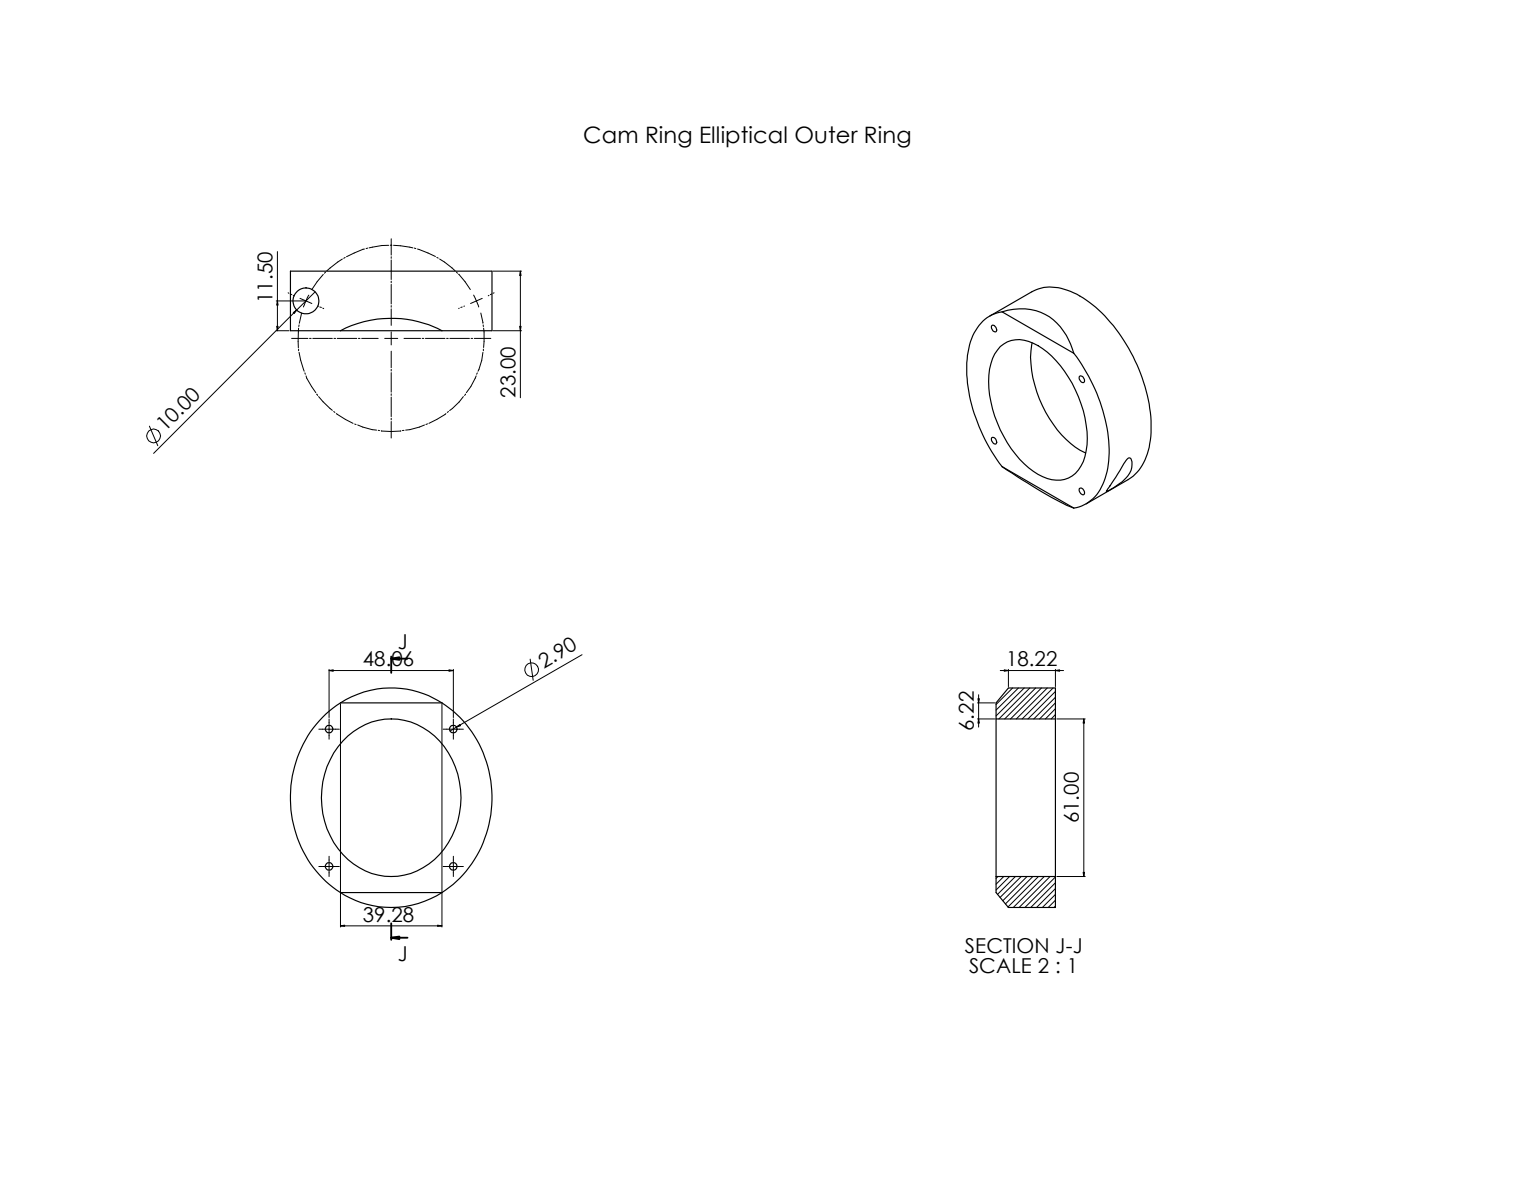
ISO-10303-21;
HEADER;
FILE_DESCRIPTION (('STEP AP214'),
    '1' );
FILE_NAME ('Cam Ring Elliptical Outer Ring.step',
    '2026-10-18T20:16:25',
    ( '' ),
    ( '' ),
    'SwSTEP 2.0',
    'SolidWorks 2025',
    '' );
FILE_SCHEMA (( 'AUTOMOTIVE_DESIGN' ));
ENDSEC;

DATA;
#6=ADVANCED_FACE ( 'NONE', ( #26858 ), #19364, .F. ) ;
#7=CARTESIAN_POINT ( 'NONE',  ( -10.18506332983503881, -29.04537757311073065, 24.50000000000000000 ) ) ;
#35=EDGE_CURVE ( 'NONE', #21045, #27073, #21273, .T. ) ;
#67=ORIENTED_EDGE ( 'NONE', *, *, #8805, .T. ) ;
#72=LINE ( 'NONE', #9585, #22578 ) ;
#83=EDGE_LOOP ( 'NONE', ( #20575, #9372 ) ) ;
#262=CARTESIAN_POINT ( 'NONE',  ( 37.01111991330344608, -13.41299137855487977, 15.98316150592440543 ) ) ;
#276=FACE_BOUND ( 'NONE', #21490, .T. ) ;
#306=CARTESIAN_POINT ( 'NONE',  ( -19.18576292979354392, -22.55620591602727742, 1.500000000000001332 ) ) ;
#358=ORIENTED_EDGE ( 'NONE', *, *, #1752, .T. ) ;
#391=DIRECTION ( 'NONE',  ( 0.000000000000000000, 0.000000000000000000, 1.000000000000000000 ) ) ;
#417=DIRECTION ( 'NONE',  ( 0.000000000000000000, -0.6368814469962913449, -0.7709617516270896864 ) ) ;
#463=CARTESIAN_POINT ( 'NONE',  ( -28.06941827521502475, 29.50589912660750969, 12.07342606168410093 ) ) ;
#502=AXIS2_PLACEMENT_3D ( 'NONE', #13971, #30353, #16313 ) ;
#521=ORIENTED_EDGE ( 'NONE', *, *, #17753, .F. ) ;
#566=AXIS2_PLACEMENT_3D ( 'NONE', #22892, #22733, #8869 ) ;
#617=EDGE_CURVE ( 'NONE', #17587, #16446, #72, .T. ) ;
#647=CARTESIAN_POINT ( 'NONE',  ( 30.67761959283033235, -26.24282937179839337, 17.43639551542309718 ) ) ;
#664=ORIENTED_EDGE ( 'NONE', *, *, #18976, .F. ) ;
#674=CARTESIAN_POINT ( 'NONE',  ( -35.78636641679163688, 16.94032250535760653, 17.18098098232441018 ) ) ;
#680=DIRECTION ( 'NONE',  ( 1.000000000000000000, 0.000000000000000000, -0.000000000000000000 ) ) ;
#716=CARTESIAN_POINT ( 'NONE',  ( 32.98805937973595093, -22.67054169308931222, 8.000000000000003553 ) ) ;
#724=DIRECTION ( 'NONE',  ( -1.000000000000000000, 0.000000000000000000, 0.000000000000000000 ) ) ;
#774=PRODUCT_DEFINITION_CONTEXT ( 'detailed design', #23710, 'design' ) ;
#782=CARTESIAN_POINT ( 'NONE',  ( -24.03057240117690441, -26.57182937991348481, 1.500000000000001332 ) ) ;
#787=ADVANCED_FACE ( 'NONE', ( #2872, #12396, #22043, #15022, #21896, #10048 ), #19557, .T. ) ;
#799=EDGE_CURVE ( 'NONE', #24988, #12790, #28615, .T. ) ;
#813=CARTESIAN_POINT ( 'NONE',  ( 32.98805937973593672, 0.000000000000000000, 18.00000000000000000 ) ) ;
#820=EDGE_LOOP ( 'NONE', ( #21441, #11766, #4890, #26992 ) ) ;
#826=CARTESIAN_POINT ( 'NONE',  ( -37.62287076735433544, 11.19774653192125591, 14.88367311033162821 ) ) ;
#857=VECTOR ( 'NONE', #15365, 1000.000000000000000 ) ;
#888=CARTESIAN_POINT ( 'NONE',  ( -12.17697269691152329, 40.41958668078866879, 21.44088211123782983 ) ) ;
#909=CARTESIAN_POINT ( 'NONE',  ( 22.58267429318971864, 26.57182937991349903, 26.54355021145562787 ) ) ;
#923=CARTESIAN_POINT ( 'NONE',  ( -29.80493885133978083, 27.41358096823880786, 9.131458560479140729 ) ) ;
#947=CARTESIAN_POINT ( 'NONE',  ( 10.18506332983505303, 29.04537757311072710, 24.50000000000000000 ) ) ;
#969=CARTESIAN_POINT ( 'NONE',  ( 30.16810946264573445, -26.93506237724814412, 17.13185035612489315 ) ) ;
#992=CARTESIAN_POINT ( 'NONE',  ( -33.31304828179383293, 22.10896115714093924, 8.000000000000005329 ) ) ;
#1038=B_SPLINE_CURVE_WITH_KNOTS ( 'NONE', 3,
 ( #18272, #27795, #6420, #16082, #4219, #6712, #9365, #28701, #30717, #14183 ),
 .UNSPECIFIED., .F., .F.,
 ( 4, 2, 2, 2, 4 ),
 ( 0.000000000000000000, 0.005347349928980100683, 0.01069469985796020657, 0.01604204978694031072, 0.02138939971592041661 ),
 .UNSPECIFIED. ) ;
#1042=DIRECTION ( 'NONE',  ( -0.000000000000000000, -1.000000000000000000, -0.000000000000000000 ) ) ;
#1119=CARTESIAN_POINT ( 'NONE',  ( 29.78864511397301484, -27.43196031439082461, 9.154089586762928832 ) ) ;
#1134=DIRECTION ( 'NONE',  ( 1.000000000000000000, 0.000000000000000000, 0.000000000000000000 ) ) ;
#1140=CARTESIAN_POINT ( 'NONE',  ( 10.18506332983505303, 29.04537757311072710, 1.500000000000000000 ) ) ;
#1141=CARTESIAN_POINT ( 'NONE',  ( -34.21431199717225979, 20.40874709909905604, 8.143388502677929353 ) ) ;
#1200=ADVANCED_FACE ( 'NONE', ( #23844 ), #2488, .F. ) ;
#1234=CARTESIAN_POINT ( 'NONE',  ( -19.64177907938615064, -36.71644397333972876, 24.50000000000000000 ) ) ;
#1267=AXIS2_PLACEMENT_3D ( 'NONE', #10644, #30128, #8758 ) ;
#1278=CARTESIAN_POINT ( 'NONE',  ( 31.30424506559346298, -25.35202612174932568, 8.284888684157436956 ) ) ;
#1298=CARTESIAN_POINT ( 'NONE',  ( -6.192647045995789412, -41.97176936070047049, 20.15864424522374065 ) ) ;
#1299=CARTESIAN_POINT ( 'NONE',  ( -37.98074266006555888, 9.653107878580014400, 13.30882976141995222 ) ) ;
#1359=AXIS2_PLACEMENT_3D ( 'NONE', #12045, #21538, #28424 ) ;
#1413=CARTESIAN_POINT ( 'NONE',  ( -10.18506332983504237, -29.04537757311072710, 1.500000000000000000 ) ) ;
#1419=( GEOMETRIC_REPRESENTATION_CONTEXT ( 3 ) GLOBAL_UNCERTAINTY_ASSIGNED_CONTEXT ( ( #17991 ) ) GLOBAL_UNIT_ASSIGNED_CONTEXT ( ( #21477, #23197, #28368 ) ) REPRESENTATION_CONTEXT ( 'NONE', 'WORKASPACE' ) );
#1422=AXIS2_PLACEMENT_3D ( 'NONE', #15991, #2089, #3991 ) ;
#1507=DIRECTION ( 'NONE',  ( 0.000000000000000000, 0.000000000000000000, -1.000000000000000000 ) ) ;
#1534=CARTESIAN_POINT ( 'NONE',  ( -25.47847050916410439, -26.57182937991348481, 24.50000000000000000 ) ) ;
#1568=CARTESIAN_POINT ( 'NONE',  ( -25.47847050916410439, -26.57182937991348481, 26.54355021145562787 ) ) ;
#1615=CARTESIAN_POINT ( 'NONE',  ( -18.94750032487069902, -37.15750911010949409, 24.13564184353800712 ) ) ;
#1683=CYLINDRICAL_SURFACE ( 'NONE', #566, 4.999999999999997335 ) ;
#1690=CARTESIAN_POINT ( 'NONE',  ( -28.54661976619838981, 28.95749706969278847, 15.30506458469658071 ) ) ;
#1697=DIRECTION ( 'NONE',  ( -0.000000000000000000, -0.000000000000000000, -1.000000000000000000 ) ) ;
#1752=EDGE_CURVE ( 'NONE', #8742, #20574, #14920, .T. ) ;
#1753=DIRECTION ( 'NONE',  ( 1.000000000000000000, 0.000000000000000000, 0.000000000000000000 ) ) ;
#1759=CARTESIAN_POINT ( 'NONE',  ( -27.75715622479468081, 2.303929616531696922E-16, 24.50000000000000000 ) ) ;
#1865=AXIS2_PLACEMENT_3D ( 'NONE', #30712, #18883, #7020 ) ;
#1895=CARTESIAN_POINT ( 'NONE',  ( 19.64177907938615064, 36.71644397333972876, 24.50000000000000000 ) ) ;
#1911=CARTESIAN_POINT ( 'NONE',  ( -25.48568755041063838, 12.36160011285429583, 24.50000000000000000 ) ) ;
#1956=CARTESIAN_POINT ( 'NONE',  ( 3.395021109945021376, 30.50000000000000000, 24.50000000000000000 ) ) ;
#1962=ORIENTED_EDGE ( 'NONE', *, *, #2846, .F. ) ;
#2032=FACE_OUTER_BOUND ( 'NONE', #19721, .T. ) ;
#2089=DIRECTION ( 'NONE',  ( 0.000000000000000000, -1.000000000000000000, 0.000000000000000000 ) ) ;
#2101=CARTESIAN_POINT ( 'NONE',  ( 14.50629223094009035, 39.46103756294984777, 22.23272703466988887 ) ) ;
#2123=ORIENTED_EDGE ( 'NONE', *, *, #24038, .F. ) ;
#2132=EDGE_CURVE ( 'NONE', #24759, #6184, #9736, .T. ) ;
#2139=CARTESIAN_POINT ( 'NONE',  ( 32.98805937973593672, 0.000000000000000000, 13.00000000000000178 ) ) ;
#2156=FACE_BOUND ( 'NONE', #12173, .T. ) ;
#2217=CARTESIAN_POINT ( 'NONE',  ( 24.03057240117691862, 26.57182937991349903, 26.54355021145562787 ) ) ;
#2302=FACE_OUTER_BOUND ( 'NONE', #17026, .T. ) ;
#2381=EDGE_CURVE ( 'NONE', #17270, #19224, #29354, .T. ) ;
#2415=CARTESIAN_POINT ( 'NONE',  ( 32.98805937973593672, 0.000000000000000000, 13.00000000000000178 ) ) ;
#2420=CARTESIAN_POINT ( 'NONE',  ( 0.000000000000000000, 36.71644397333972165, 24.50000000000000000 ) ) ;
#2488=CYLINDRICAL_SURFACE ( 'NONE', #20811, 1.447898107987198646 ) ;
#2505=CARTESIAN_POINT ( 'NONE',  ( -25.48568755041063838, 12.36160011285429583, 24.50000000000000000 ) ) ;
#2608=CARTESIAN_POINT ( 'NONE',  ( 36.63885979765411349, -14.57625097221031751, 16.42869143197607684 ) ) ;
#2614=ORIENTED_EDGE ( 'NONE', *, *, #22128, .T. ) ;
#2732=DIRECTION ( 'NONE',  ( 1.000000000000000000, 0.000000000000000000, 0.000000000000000000 ) ) ;
#2765=CARTESIAN_POINT ( 'NONE',  ( 37.87340355726868779, -10.14209321046124934, 14.07067178332522239 ) ) ;
#2798=CARTESIAN_POINT ( 'NONE',  ( -30.18521284010790851, 26.91230962269908034, 8.856508891382476989 ) ) ;
#2846=EDGE_CURVE ( 'NONE', #25535, #4436, #15712, .T. ) ;
#2854=DIRECTION ( 'NONE',  ( -0.000000000000000000, -0.000000000000000000, -1.000000000000000000 ) ) ;
#2872=FACE_BOUND ( 'NONE', #7887, .T. ) ;
#2919=CARTESIAN_POINT ( 'NONE',  ( -22.58267429318971864, 26.57182937991348481, 26.54355021145562787 ) ) ;
#2939=ORIENTED_EDGE ( 'NONE', *, *, #28576, .F. ) ;
#2966=CARTESIAN_POINT ( 'NONE',  ( -28.10697575488836364, 29.46351030971690932, 14.10614635148330898 ) ) ;
#3002=CARTESIAN_POINT ( 'NONE',  ( 29.54181686732680845, -27.74713163033052865, 9.373611838719332567 ) ) ;
#3016=EDGE_LOOP ( 'NONE', ( #29920, #15554 ) ) ;
#3031=DIRECTION ( 'NONE',  ( 0.000000000000000000, 0.000000000000000000, 1.000000000000000000 ) ) ;
#3068=PLANE ( 'NONE',  #24267 ) ;
#3069=CARTESIAN_POINT ( 'NONE',  ( 37.79362409831109915, -10.49224821554092735, 11.60540311995022833 ) ) ;
#3151=CARTESIAN_POINT ( 'NONE',  ( 30.28907500942318620, -26.77591773196712310, 8.779599968084907502 ) ) ;
#3173=DIRECTION ( 'NONE',  ( 1.000000000000000000, 0.000000000000000000, 0.000000000000000000 ) ) ;
#3177=CARTESIAN_POINT ( 'NONE',  ( -37.98866957712698422, 9.615774924837397819, 13.14437204739174447 ) ) ;
#3216=CARTESIAN_POINT ( 'NONE',  ( -3.469446951953614189E-15, -30.50000000000000711, 1.500000000000000000 ) ) ;
#3220=CARTESIAN_POINT ( 'NONE',  ( 37.66982319287888004, -11.00826088415979775, 11.23380626198473387 ) ) ;
#3225=ORIENTED_EDGE ( 'NONE', *, *, #3454, .F. ) ;
#3227=CARTESIAN_POINT ( 'NONE',  ( -7.114862909856333850, 41.83185039483213075, 20.27422947789757046 ) ) ;
#3228=CARTESIAN_POINT ( 'NONE',  ( -48.64405085385531180, 18.29172496293576344, 24.50000000000000355 ) ) ;
#3252=CARTESIAN_POINT ( 'NONE',  ( -32.98805937973593672, 22.67054169308932288, 8.000000000000003553 ) ) ;
#3277=CARTESIAN_POINT ( 'NONE',  ( 25.48568755041062417, 12.36160011285428872, 1.500000000000001332 ) ) ;
#3324=CARTESIAN_POINT ( 'NONE',  ( 10.18506332983503349, -29.04537757311073420, 1.500000000000000000 ) ) ;
#3325=CARTESIAN_POINT ( 'NONE',  ( -37.98737094879278686, 9.621865500938454829, 12.81607210702588340 ) ) ;
#3358=ORIENTED_EDGE ( 'NONE', *, *, #26402, .F. ) ;
#3438=DIRECTION ( 'NONE',  ( 0.000000000000000000, 0.000000000000000000, 1.000000000000000000 ) ) ;
#3440=CARTESIAN_POINT ( 'NONE',  ( 3.469446951953614189E-15, 30.50000000000000000, 24.50000000000000000 ) ) ;
#3454=EDGE_CURVE ( 'NONE', #16680, #16446, #9263, .T. ) ;
#3482=CARTESIAN_POINT ( 'NONE',  ( 24.03057240117690441, -26.57182937991349903, 1.500000000000001332 ) ) ;
#3489=CARTESIAN_POINT ( 'NONE',  ( 25.48568755041062417, 12.36160011285428872, 1.500000000000000000 ) ) ;
#3543=VERTEX_POINT ( 'NONE', #10112 ) ;
#3597=VERTEX_POINT ( 'NONE', #22890 ) ;
#3640=CARTESIAN_POINT ( 'NONE',  ( -37.48217255283579874, 11.74471995787475187, 15.19832840420940734 ) ) ;
#3646=CARTESIAN_POINT ( 'NONE',  ( 2.168404344971008868E-16, 30.50000000000000000, 24.50000000000000000 ) ) ;
#3698=CARTESIAN_POINT ( 'NONE',  ( 22.58267429318970443, -26.57182937991349903, 26.54355021145562787 ) ) ;
#3701=ADVANCED_FACE ( 'NONE', ( #18676 ), #20697, .F. ) ;
#3759=( BOUNDED_SURFACE ( )  B_SPLINE_SURFACE ( 3, 1, ( 
 ( #4545, #13914 ),
 ( #6734, #16245 ),
 ( #25916, #11431 ),
 ( #4855, #16401 ) ),
 .UNSPECIFIED., .F., .F., .T. ) 
 B_SPLINE_SURFACE_WITH_KNOTS ( ( 4, 4 ),
 ( 2, 2 ),
 ( 0.000000000000000000, 1.000000000000000000 ),
 ( 0.000000000000000000, 1.000000000000000000 ),
 .UNSPECIFIED. ) 
 GEOMETRIC_REPRESENTATION_ITEM ( )  RATIONAL_B_SPLINE_SURFACE ( (
 ( 1.000000000000000000, 1.000000000000000000),
 ( 0.3333333333333333703, 0.3333333333333333703),
 ( 0.3333333333333333703, 0.3333333333333333703),
 ( 1.000000000000000000, 1.000000000000000000) ) ) 
 REPRESENTATION_ITEM ( '' )  SURFACE ( )  );
#3881=EDGE_CURVE ( 'NONE', #8417, #14704, #23959, .T. ) ;
#3883=CARTESIAN_POINT ( 'NONE',  ( -22.58267429318970443, -26.57182937991348481, 26.54355021145562787 ) ) ;
#3889=CARTESIAN_POINT ( 'NONE',  ( -29.41946345040754096, 27.90099610680150377, 16.50653305109835500 ) ) ;
#3912=FACE_OUTER_BOUND ( 'NONE', #27376, .T. ) ;
#3970=B_SPLINE_CURVE_WITH_KNOTS ( 'NONE', 3,
 ( #19233, #18949, #16589, #19088, #4896, #19696, #674, #10502, #8494, #25001, #13156, #22037, #3640, #826, #10350, #29221, #29532, #20328, #7860, #1299, #3177, #3325, #12856, #17369, #29853, #22648, #24683, #22495, #24531, #27043, #15483, #19862, #10814, #20163, #29380, #8020, #8169, #17522, #1141, #5824, #992, #26729 ),
 .UNSPECIFIED., .F., .F.,
 ( 4, 2, 2, 2, 2, 2, 2, 2, 2, 2, 2, 2, 2, 2, 2, 2, 2, 2, 2, 2, 4 ),
 ( 0.02151600789256482779, 0.02343308447725669583, 0.02535016106194856386, 0.02918431423133229299, 0.03110139081602415062, 0.03301846740071601172, 0.03397700569306194573, 0.03493554398540787975, 0.03589408227775381377, 0.03637335142392678078, 0.03685262057009974779, 0.03733188971627271480, 0.03781115886244568874, 0.03876969715479162970, 0.03972823544713757066, 0.04068677373948351161, 0.04260385032417539353, 0.04452092690886727544, 0.04835508007825103927, 0.05027215666294292118, 0.05218923324763480309 ),
 .UNSPECIFIED. ) ;
#3991=DIRECTION ( 'NONE',  ( 0.000000000000000000, 0.000000000000000000, 1.000000000000000000 ) ) ;
#4029=FACE_OUTER_BOUND ( 'NONE', #6532, .T. ) ;
#4056=ORIENTED_EDGE ( 'NONE', *, *, #35, .F. ) ;
#4135=PLANE ( 'NONE',  #1422 ) ;
#4150=CARTESIAN_POINT ( 'NONE',  ( -19.64177907938615064, -36.71644397333972876, 24.50000000000000000 ) ) ;
#4207=EDGE_CURVE ( 'NONE', #12790, #24988, #12731, .T. ) ;
#4219=CARTESIAN_POINT ( 'NONE',  ( 12.13957942244085331, -40.43335259791965086, 21.42951026665136993 ) ) ;
#4238=CIRCLE ( 'NONE', #1267, 1.447898107987198646 ) ;
#4346=EDGE_LOOP ( 'NONE', ( #5689, #11400, #10833, #14682 ) ) ;
#4354=CARTESIAN_POINT ( 'NONE',  ( 22.58267429318970443, -26.57182937991349903, 24.50000000000000000 ) ) ;
#4429=ADVANCED_FACE ( 'NONE', ( #18306 ), #16112, .F. ) ;
#4436=VERTEX_POINT ( 'NONE', #11440 ) ;
#4502=VERTEX_POINT ( 'NONE', #27662 ) ;
#4520=CARTESIAN_POINT ( 'NONE',  ( 32.98805937973592961, -22.67054169308934064, 18.00000000000000000 ) ) ;
#4545=CARTESIAN_POINT ( 'NONE',  ( -4.776122516674677878E-15, -42.50000000000000000, 24.50000000000000000 ) ) ;
#4781=CARTESIAN_POINT ( 'NONE',  ( 34.23529990058388250, -20.39752770391714876, 17.87601422035457333 ) ) ;
#4789=ORIENTED_EDGE ( 'NONE', *, *, #24819, .F. ) ;
#4848=UNCERTAINTY_MEASURE_WITH_UNIT (LENGTH_MEASURE( 1.000000000000000082E-05 ), #21403, 'distance_accuracy_value', 'NONE');
#4854=AXIS2_PLACEMENT_3D ( 'NONE', #29179, #19979, #7517 ) ;
#4855=CARTESIAN_POINT ( 'NONE',  ( 0.000000000000000000, 42.50000000000000000, 24.50000000000000000 ) ) ;
#4871=CARTESIAN_POINT ( 'NONE',  ( -22.58267429318970443, -26.57182937991348481, 24.50000000000000000 ) ) ;
#4890=ORIENTED_EDGE ( 'NONE', *, *, #3454, .T. ) ;
#4896=CARTESIAN_POINT ( 'NONE',  ( -34.50378612593421224, 19.82132163181573148, 17.77334831411353733 ) ) ;
#4913=ORIENTED_EDGE ( 'NONE', *, *, #16059, .F. ) ;
#4915=CARTESIAN_POINT ( 'NONE',  ( -3.469446951953614189E-15, -30.50000000000000711, 24.50000000000000000 ) ) ;
#4947=CARTESIAN_POINT ( 'NONE',  ( 37.94146307560947662, -9.835134691610786462, 13.69354701980937961 ) ) ;
#4961=FACE_BOUND ( 'NONE', #30357, .T. ) ;
#5020=CYLINDRICAL_SURFACE ( 'NONE', #1359, 1.447898107987198646 ) ;
#5032=ADVANCED_FACE ( 'NONE', ( #8064 ), #3068, .F. ) ;
#5038=CIRCLE ( 'NONE', #21514, 1.447898107987198646 ) ;
#5040=AXIS2_PLACEMENT_3D ( 'NONE', #16169, #25068, #25684 ) ;
#5077=CYLINDRICAL_SURFACE ( 'NONE', #10597, 1.447898107987198646 ) ;
#5133=ORIENTED_EDGE ( 'NONE', *, *, #13621, .T. ) ;
#5150=CARTESIAN_POINT ( 'NONE',  ( 24.03057240117690441, -26.57182937991349903, 24.50000000000000000 ) ) ;
#5199=PRODUCT ( 'Cam Ring Elliptical Outer Ring', 'Cam Ring Elliptical Outer Ring', '', ( #24403 ) ) ;
#5204=ADVANCED_FACE ( 'NONE', ( #5871 ), #23001, .F. ) ;
#5207=CARTESIAN_POINT ( 'NONE',  ( -3.469446951953614189E-15, -30.50000000000000711, 1.500000000000000000 ) ) ;
#5235=CARTESIAN_POINT ( 'NONE',  ( -22.58267429318970443, -26.57182937991348481, 1.500000000000001332 ) ) ;
#5256=CARTESIAN_POINT ( 'NONE',  ( 37.70070167288648122, -10.88189949536004342, 14.68280373647734116 ) ) ;
#5278=ORIENTED_EDGE ( 'NONE', *, *, #25507, .F. ) ;
#5290=CARTESIAN_POINT ( 'NONE',  ( -28.00213357088913924, 29.58171923439856243, 13.43815007647722659 ) ) ;
#5316=CARTESIAN_POINT ( 'NONE',  ( 77.99999999999998579, 42.50000000000000000, 1.500000000000000222 ) ) ;
#5332=CARTESIAN_POINT ( 'NONE',  ( 28.30074574513791674, -29.24255319736864323, 14.75302129891823988 ) ) ;
#5363=ORIENTED_EDGE ( 'NONE', *, *, #24082, .F. ) ;
#5455=CARTESIAN_POINT ( 'NONE',  ( -28.29454325412426030, 29.24967321222531780, 14.73627230915420583 ) ) ;
#5493=CARTESIAN_POINT ( 'NONE',  ( 32.52407683584942788, -23.45431533902839405, 17.97980913012589710 ) ) ;
#5574=CARTESIAN_POINT ( 'NONE',  ( -8.074094344234884818E-15, 42.50000000000000000, 19.72227980406325543 ) ) ;
#5600=B_SPLINE_CURVE_WITH_KNOTS ( 'NONE', 3,
 ( #16648, #26154, #4781, #23805, #24576, #8065, #12126, #17570, #2608, #262, #19745, #14756, #15062, #22082, #5256, #7448, #21781, #2765, #7597, #4947, #19446, #26943, #24428, #12592, #21627, #28962, #26789, #19918, #24276, #12278, #3069, #3220, #24116, #19292, #29432, #9775, #14459, #28811, #23961, #21934, #22242, #7916, #16951, #716 ),
 .UNSPECIFIED., .F., .F.,
 ( 4, 2, 2, 2, 2, 2, 2, 2, 2, 2, 2, 2, 2, 2, 2, 2, 2, 2, 2, 2, 2, 4 ),
 ( 6.938893903907228378E-18, 0.003866689226559128639, 0.005800033839838692959, 0.007733378453118257279, 0.009666723066397821598, 0.01160006767967738592, 0.01256673998631717241, 0.01353341229295695718, 0.01401674844627684956, 0.01450008459959674367, 0.01498342075291663779, 0.01522508882957658398, 0.01546675690623653190, 0.01595009305955642429, 0.01643342921287630973, 0.01740010151951609102, 0.01836677382615587231, 0.01933344613279565360, 0.02126679074607521619, 0.02320013535935478224, 0.02706682458591391088, 0.03093351381247303605 ),
 .UNSPECIFIED. ) ;
#5632=CARTESIAN_POINT ( 'NONE',  ( 19.18576292979354392, -22.55620591602728453, 1.500000000000001332 ) ) ;
#5689=ORIENTED_EDGE ( 'NONE', *, *, #25026, .F. ) ;
#5720=CARTESIAN_POINT ( 'NONE',  ( 24.03057240117690441, -26.57182937991349903, 26.54355021145562787 ) ) ;
#5730=ADVANCED_FACE ( 'NONE', ( #30600 ), #27828, .F. ) ;
#5762=ORIENTED_EDGE ( 'NONE', *, *, #20655, .F. ) ;
#5824=CARTESIAN_POINT ( 'NONE',  ( -33.62358953728911359, 21.54311338121501507, 8.031451707336353607 ) ) ;
#5853=CARTESIAN_POINT ( 'NONE',  ( -32.98805937973593672, 0.000000000000000000, 18.00000000000000000 ) ) ;
#5865=CARTESIAN_POINT ( 'NONE',  ( -32.98805937973593672, 80.00000000000000000, 8.000000000000003553 ) ) ;
#5871=FACE_OUTER_BOUND ( 'NONE', #7763, .T. ) ;
#5933=ORIENTED_EDGE ( 'NONE', *, *, #18705, .F. ) ;
#5983=DIRECTION ( 'NONE',  ( 0.000000000000000000, 0.000000000000000000, 1.000000000000000000 ) ) ;
#6062=CARTESIAN_POINT ( 'NONE',  ( -32.05743189141918492, 24.22168755390175576, 17.93996624350626590 ) ) ;
#6126=CARTESIAN_POINT ( 'NONE',  ( -12.13118772005164026, -40.43574026512624897, 21.42753784591547017 ) ) ;
#6184=VERTEX_POINT ( 'NONE', #27241 ) ;
#6236=CARTESIAN_POINT ( 'NONE',  ( 24.03057240117690441, -26.57182937991349903, 1.500000000000001332 ) ) ;
#6346=DIRECTION ( 'NONE',  ( 0.000000000000000000, -1.000000000000000000, 0.000000000000000000 ) ) ;
#6364=CIRCLE ( 'NONE', #26278, 1.447898107987198646 ) ;
#6380=CARTESIAN_POINT ( 'NONE',  ( -29.78995557804746497, 27.43027642362437390, 16.84702627303446221 ) ) ;
#6420=CARTESIAN_POINT ( 'NONE',  ( 16.79415820840736728, -38.40031270401642871, 23.10897800509315658 ) ) ;
#6426=CIRCLE ( 'NONE', #8442, 4.999999999999997335 ) ;
#6439=MECHANICAL_DESIGN_GEOMETRIC_PRESENTATION_REPRESENTATION('',(#19881),#14397);
#6444=CARTESIAN_POINT ( 'NONE',  ( -4.776122516674677878E-15, -42.50000000000000000, 19.72227980406325543 ) ) ;
#6498=ORIENTED_EDGE ( 'NONE', *, *, #26501, .T. ) ;
#6532=EDGE_LOOP ( 'NONE', ( #22804, #521, #30469, #26719 ) ) ;
#6555=ORIENTED_EDGE ( 'NONE', *, *, #2132, .T. ) ;
#6633=CARTESIAN_POINT ( 'NONE',  ( 10.18506332983503349, -29.04537757311073420, 24.50000000000000000 ) ) ;
#6712=CARTESIAN_POINT ( 'NONE',  ( 8.778767752581492445, -41.45290410434266448, 20.58727206569324153 ) ) ;
#6723=CARTESIAN_POINT ( 'NONE',  ( 19.64177907938615064, -36.71644397333972876, 24.50000000000000000 ) ) ;
#6734=CARTESIAN_POINT ( 'NONE',  ( 77.99999999999998579, -42.50000000000002132, 24.50000000000000000 ) ) ;
#6782=CARTESIAN_POINT ( 'NONE',  ( 1.794035659141604899, 42.46622758119957552, 19.75017875872448059 ) ) ;
#6789=FACE_OUTER_BOUND ( 'NONE', #820, .T. ) ;
#6801=VECTOR ( 'NONE', #27037, 1000.000000000000000 ) ;
#6845=PRODUCT_DEFINITION ( 'UNKNOWN', '', #8918, #774 ) ;
#6900=VECTOR ( 'NONE', #17424, 1000.000000000000000 ) ;
#7020=DIRECTION ( 'NONE',  ( -1.000000000000000000, 0.000000000000000000, 0.000000000000000000 ) ) ;
#7031=ORIENTED_EDGE ( 'NONE', *, *, #21011, .F. ) ;
#7175=CARTESIAN_POINT ( 'NONE',  ( 0.000000000000000000, 42.50000000000000000, 24.50000000000000000 ) ) ;
#7212=( NAMED_UNIT ( * ) PLANE_ANGLE_UNIT ( ) SI_UNIT ( $, .RADIAN. ) );
#7245=EDGE_CURVE ( 'NONE', #3543, #29877, #21049, .T. ) ;
#7344=CARTESIAN_POINT ( 'NONE',  ( -19.18576292979354392, -22.55620591602727742, 24.50000000000000000 ) ) ;
#7349=DIRECTION ( 'NONE',  ( 0.000000000000000000, 0.000000000000000000, 1.000000000000000000 ) ) ;
#7368=ORIENTED_EDGE ( 'NONE', *, *, #29806, .F. ) ;
#7396=AXIS2_PLACEMENT_3D ( 'NONE', #9486, #28514, #21014 ) ;
#7448=CARTESIAN_POINT ( 'NONE',  ( 37.79101548699587454, -10.50083399009356988, 14.39349168688145575 ) ) ;
#7498=CARTESIAN_POINT ( 'NONE',  ( -3.395021109945006721, -30.50000000000000711, 1.500000000000001332 ) ) ;
#7517=DIRECTION ( 'NONE',  ( 0.000000000000000000, 0.7709617516270895754, 0.6368814469962912339 ) ) ;
#7597=CARTESIAN_POINT ( 'NONE',  ( 37.89827105978137922, -10.03094553435206926, 13.95238484874844787 ) ) ;
#7634=CARTESIAN_POINT ( 'NONE',  ( -27.98709118423092690, 29.59858197539721658, 13.20579471836786745 ) ) ;
#7641=ADVANCED_FACE ( 'NONE', ( #26447 ), #5077, .F. ) ;
#7660=VECTOR ( 'NONE', #18726, 1000.000000000000000 ) ;
#7682=CARTESIAN_POINT ( 'NONE',  ( 27.98837345756654926, -29.59714202224856194, 13.23495098233264500 ) ) ;
#7688=EDGE_CURVE ( 'NONE', #26441, #20574, #18128, .T. ) ;
#7763=EDGE_LOOP ( 'NONE', ( #29336, #358, #5133, #5933 ) ) ;
#7782=CARTESIAN_POINT ( 'NONE',  ( -24.03057240117691862, 26.57182937991348481, 24.50000000000000000 ) ) ;
#7831=CARTESIAN_POINT ( 'NONE',  ( 32.40545545705547426, -23.64849546015198811, 17.96741959276885581 ) ) ;
#7837=AXIS2_PLACEMENT_3D ( 'NONE', #11186, #22716, #27884 ) ;
#7860=CARTESIAN_POINT ( 'NONE',  ( -37.95344354766306338, 9.779784673403119299, 13.60598863365600053 ) ) ;
#7864=DIRECTION ( 'NONE',  ( -0.000000000000000000, 1.000000000000000000, -0.000000000000000000 ) ) ;
#7887=EDGE_LOOP ( 'NONE', ( #5363, #4056 ) ) ;
#7916=CARTESIAN_POINT ( 'NONE',  ( 34.22030469044062073, -20.42639397296790804, 8.120957071897569435 ) ) ;
#7926=FACE_OUTER_BOUND ( 'NONE', #16867, .T. ) ;
#7952=DIRECTION ( 'NONE',  ( 1.000000000000000000, 0.000000000000000000, 0.000000000000000000 ) ) ;
#7998=CARTESIAN_POINT ( 'NONE',  ( 28.11261193835277084, -29.45712586627402985, 14.13030833143228371 ) ) ;
#8019=CARTESIAN_POINT ( 'NONE',  ( 27.75715622479469147, -6.315477654728063328E-15, 1.500000000000000000 ) ) ;
#8020=CARTESIAN_POINT ( 'NONE',  ( -35.77650053662277685, 16.96546617299160076, 8.812125201147090081 ) ) ;
#8059=LINE ( 'NONE', #5865, #857 ) ;
#8064=FACE_OUTER_BOUND ( 'NONE', #12470, .T. ) ;
#8065=CARTESIAN_POINT ( 'NONE',  ( 35.77999848792182291, -16.92214645512589755, 17.15740857515053364 ) ) ;
#8076=CYLINDRICAL_SURFACE ( 'NONE', #14140, 1.447898107987198646 ) ;
#8105=CARTESIAN_POINT ( 'NONE',  ( -30.31362811597099238, 26.74039424657907205, 8.772790042427574875 ) ) ;
#8119=B_SPLINE_CURVE_WITH_KNOTS ( 'NONE', 3,
 ( #15570, #28153, #6782, #10741, #13964, #20823, #23460, #17761, #8986, #23318, #2101, #18502, #11623, #18802 ),
 .UNSPECIFIED., .F., .F.,
 ( 4, 2, 2, 2, 2, 2, 4 ),
 ( 0.02129242833620984335, 0.02395618414067833199, 0.02661993994514682063, 0.03194745155408380138, 0.03461120735855229003, 0.03727496316302077867, 0.04260247477195776289 ),
 .UNSPECIFIED. ) ;
#8127=DIRECTION ( 'NONE',  ( -0.000000000000000000, -0.000000000000000000, -1.000000000000000000 ) ) ;
#8147=CARTESIAN_POINT ( 'NONE',  ( 31.04966398092921409, -25.72093259340003968, 8.382396669768365172 ) ) ;
#8169=CARTESIAN_POINT ( 'NONE',  ( -35.29666319828150023, 18.12171425783904866, 8.528199801003413683 ) ) ;
#8330=CARTESIAN_POINT ( 'NONE',  ( 32.98805937973593672, -80.00000000000000000, 13.00000000000000178 ) ) ;
#8344=ORIENTED_EDGE ( 'NONE', *, *, #15087, .T. ) ;
#8389=DIRECTION ( 'NONE',  ( 0.000000000000000000, 0.000000000000000000, 1.000000000000000000 ) ) ;
#8407=B_SPLINE_SURFACE_WITH_KNOTS ( 'NONE', 3, 1, ( 
 ( #20125, #29956 ),
 ( #29805, #17482 ),
 ( #13271, #27004 ),
 ( #15272, #5632 ),
 ( #24803, #29643 ),
 ( #15127, #8448 ),
 ( #24643, #3277 ),
 ( #17791, #12806 ),
 ( #947, #10459 ),
 ( #19973, #29492 ),
 ( #3440, #12961 ) ),
 .UNSPECIFIED., .F., .F., .F.,
 ( 4, 1, 1, 1, 1, 1, 1, 1, 4 ),
 ( 2, 2 ),
 ( 3.141592653589793116, 3.534291735288517255, 3.926990816987241395, 4.319689898685965090, 4.712388980384689674, 5.105088062083414258, 5.497787143782137953, 5.890486225480861648, 6.283185307179586232 ),
 ( 0.000000000000000000, 1.000000000000000000 ),
 .UNSPECIFIED. ) ;
#8417=VERTEX_POINT ( 'NONE', #9350 ) ;
#8442=AXIS2_PLACEMENT_3D ( 'NONE', #20677, #6346, #8389 ) ;
#8448=CARTESIAN_POINT ( 'NONE',  ( 27.75715622479469147, -6.315477654728063328E-15, 1.500000000000001332 ) ) ;
#8452=EDGE_CURVE ( 'NONE', #17270, #16132, #18072, .T. ) ;
#8458=CIRCLE ( 'NONE', #11942, 1.447898107987198646 ) ;
#8471=ADVANCED_FACE ( 'NONE', ( #4029 ), #1683, .F. ) ;
#8479=ORIENTED_EDGE ( 'NONE', *, *, #22585, .T. ) ;
#8494=CARTESIAN_POINT ( 'NONE',  ( -36.62615482024158098, 14.61410224498927946, 16.44210843200423255 ) ) ;
#8522=VERTEX_POINT ( 'NONE', #1234 ) ;
#8550=VERTEX_POINT ( 'NONE', #17925 ) ;
#8555=CARTESIAN_POINT ( 'NONE',  ( -19.64177907938615064, 36.71644397333972876, 24.50000000000000000 ) ) ;
#8568=DIRECTION ( 'NONE',  ( -0.000000000000000000, -0.000000000000000000, -1.000000000000000000 ) ) ;
#8583=CARTESIAN_POINT ( 'NONE',  ( 2.168404344971008868E-16, 30.50000000000000000, 1.500000000000000000 ) ) ;
#8639=CARTESIAN_POINT ( 'NONE',  ( -3.395021109945014270, 30.50000000000000355, 24.50000000000000000 ) ) ;
#8678=CARTESIAN_POINT ( 'NONE',  ( -3.469446951953614189E-15, -30.50000000000000711, 24.50000000000000000 ) ) ;
#8742=VERTEX_POINT ( 'NONE', #23960 ) ;
#8758=DIRECTION ( 'NONE',  ( 1.000000000000000000, 0.000000000000000000, 0.000000000000000000 ) ) ;
#8771=CARTESIAN_POINT ( 'NONE',  ( -13.72594918703051725, -39.82203247533167456, 21.93451384618056110 ) ) ;
#8791=B_SPLINE_CURVE_WITH_KNOTS ( 'NONE', 3,
 ( #6444, #20620, #11432, #1298, #22960, #20476, #27964, #6126, #8771, #8942, #27654, #17997, #1615, #25475 ),
 .UNSPECIFIED., .F., .F.,
 ( 4, 2, 2, 2, 2, 2, 4 ),
 ( 0.02138939971592041661, 0.02672123144516384136, 0.02938714730978555373, 0.03205306317440725916, 0.03738489490365068391, 0.04005081076827241016, 0.04271672663289412947 ),
 .UNSPECIFIED. ) ;
#8805=EDGE_CURVE ( 'NONE', #9785, #6184, #8119, .T. ) ;
#8825=CARTESIAN_POINT ( 'NONE',  ( 3.395021109945009385, -30.50000000000000711, 24.50000000000000000 ) ) ;
#8826=CARTESIAN_POINT ( 'NONE',  ( -32.98805937973593672, 80.00000000000000000, 13.00000000000000178 ) ) ;
#8869=DIRECTION ( 'NONE',  ( 0.000000000000000000, 0.000000000000000000, -1.000000000000000000 ) ) ;
#8914=ORIENTED_EDGE ( 'NONE', *, *, #2381, .F. ) ;
#8918=PRODUCT_DEFINITION_FORMATION_WITH_SPECIFIED_SOURCE ( 'ANY', '', #5199, .NOT_KNOWN. ) ;
#8942=CARTESIAN_POINT ( 'NONE',  ( -16.01986981312618852, -38.75956249542284127, 22.81220643827916561 ) ) ;
#8948=CARTESIAN_POINT ( 'NONE',  ( -19.18576292979354037, 22.55620591602727387, 24.50000000000000000 ) ) ;
#8974=ORIENTED_EDGE ( 'NONE', *, *, #4207, .F. ) ;
#8986=CARTESIAN_POINT ( 'NONE',  ( 12.11357906259289230, 40.40859726677000197, 21.44996032281847320 ) ) ;
#9008=ORIENTED_EDGE ( 'NONE', *, *, #21011, .T. ) ;
#9115=CARTESIAN_POINT ( 'NONE',  ( -8.074094344234884818E-15, 42.50000000000000000, 19.72227980406325543 ) ) ;
#9162=EDGE_CURVE ( 'NONE', #3597, #17587, #22605, .T. ) ;
#9207=CARTESIAN_POINT ( 'NONE',  ( -4.776122516674677878E-15, -42.50000000000000000, 1.500000000000001332 ) ) ;
#9211=CARTESIAN_POINT ( 'NONE',  ( -25.47847050916411504, 26.57182937991348481, 26.54355021145562787 ) ) ;
#9263=CIRCLE ( 'NONE', #12252, 4.999999999999997335 ) ;
#9314=CIRCLE ( 'NONE', #25746, 1.447898107987198646 ) ;
#9350=CARTESIAN_POINT ( 'NONE',  ( -22.58267429318971864, 26.57182937991348481, 24.50000000000000000 ) ) ;
#9365=CARTESIAN_POINT ( 'NONE',  ( 7.067645071111839705, -41.84023411754124311, 20.26730379392047610 ) ) ;
#9372=ORIENTED_EDGE ( 'NONE', *, *, #9162, .T. ) ;
#9391=DIRECTION ( 'NONE',  ( -0.000000000000000000, -0.000000000000000000, -1.000000000000000000 ) ) ;
#9394=ADVANCED_FACE ( 'NONE', ( #2032, #11556 ), #25253, .F. ) ;
#9409=ADVANCED_FACE ( 'NONE', ( #14343 ), #21359, .F. ) ;
#9486=CARTESIAN_POINT ( 'NONE',  ( 0.000000000000000000, 0.000000000000000000, 0.000000000000000000 ) ) ;
#9513=CARTESIAN_POINT ( 'NONE',  ( 0.000000000000000000, 42.50000000000000000, 1.500000000000001332 ) ) ;
#9531=EDGE_LOOP ( 'NONE', ( #27762, #2614, #14193, #10948 ) ) ;
#9585=CARTESIAN_POINT ( 'NONE',  ( 32.98805937973593672, -80.00000000000000000, 18.00000000000000000 ) ) ;
#9665=EDGE_LOOP ( 'NONE', ( #16469, #8914 ) ) ;
#9718=ORIENTED_EDGE ( 'NONE', *, *, #26543, .F. ) ;
#9736=LINE ( 'NONE', #2420, #24350 ) ;
#9764=CARTESIAN_POINT ( 'NONE',  ( 25.47847050916411504, 26.57182937991349903, 1.500000000000001332 ) ) ;
#9772=AXIS2_PLACEMENT_3D ( 'NONE', #2139, #16181, #30666 ) ;
#9775=CARTESIAN_POINT ( 'NONE',  ( 37.14925617980244255, -12.95022789879826419, 10.21045242721227275 ) ) ;
#9785=VERTEX_POINT ( 'NONE', #9115 ) ;
#9787=CARTESIAN_POINT ( 'NONE',  ( -18.25679605800083749, 37.59630342716597795, 23.77315958162180465 ) ) ;
#9818=CARTESIAN_POINT ( 'NONE',  ( -31.32177610871843854, 25.32617988875603032, 8.278890997040555533 ) ) ;
#9830=CARTESIAN_POINT ( 'NONE',  ( -3.395021109945014270, 30.50000000000000355, 24.50000000000000000 ) ) ;
#9934=AXIS2_PLACEMENT_3D ( 'NONE', #23932, #14884, #2732 ) ;
#10039=CARTESIAN_POINT ( 'NONE',  ( 24.03057240117691862, 26.57182937991349903, 24.50000000000000000 ) ) ;
#10048=FACE_BOUND ( 'NONE', #13149, .T. ) ;
#10091=CARTESIAN_POINT ( 'NONE',  ( -0.8974428369466271871, 42.49999999999999289, 19.72227980406326253 ) ) ;
#10112=CARTESIAN_POINT ( 'NONE',  ( -25.47847050916411504, 26.57182937991348481, 24.50000000000000000 ) ) ;
#10156=ORIENTED_EDGE ( 'NONE', *, *, #18537, .T. ) ;
#10162=CARTESIAN_POINT ( 'NONE',  ( 31.05675150279763130, -25.71074496668444098, 17.62049765687706682 ) ) ;
#10165=EDGE_CURVE ( 'NONE', #12790, #10393, #16405, .T. ) ;
#10178=ORIENTED_EDGE ( 'NONE', *, *, #28576, .T. ) ;
#10241=CARTESIAN_POINT ( 'NONE',  ( -4.468018643628994369, 42.23132757233521772, 19.94422659213416082 ) ) ;
#10303=CARTESIAN_POINT ( 'NONE',  ( -4.776122516674677878E-15, -42.50000000000000000, 19.72227980406325543 ) ) ;
#10318=CARTESIAN_POINT ( 'NONE',  ( 29.06906351934491184, -28.33367601428275151, 9.889412824572042737 ) ) ;
#10350=CARTESIAN_POINT ( 'NONE',  ( -37.68891294954676141, 10.93031833424447363, 14.71512993969763450 ) ) ;
#10393=VERTEX_POINT ( 'NONE', #3216 ) ;
#10445=CARTESIAN_POINT ( 'NONE',  ( -22.58267429318971864, 26.57182937991348481, 1.500000000000001332 ) ) ;
#10459=CARTESIAN_POINT ( 'NONE',  ( 10.18506332983505303, 29.04537757311072710, 1.500000000000001332 ) ) ;
#10478=CARTESIAN_POINT ( 'NONE',  ( 28.55449552082023601, -28.94826332574320560, 15.31987994115628737 ) ) ;
#10499=DIRECTION ( 'NONE',  ( 0.000000000000000000, 0.000000000000000000, 1.000000000000000000 ) ) ;
#10502=CARTESIAN_POINT ( 'NONE',  ( -36.42579814062143129, 15.19756091628274319, 16.64139166720004326 ) ) ;
#10597=AXIS2_PLACEMENT_3D ( 'NONE', #14589, #1697, #11781 ) ;
#10608=CARTESIAN_POINT ( 'NONE',  ( -3.469446951953614189E-15, -30.50000000000000711, 1.500000000000000000 ) ) ;
#10631=CARTESIAN_POINT ( 'NONE',  ( 28.74414854879570314, -28.72450863477462235, 10.34889633708970536 ) ) ;
#10633=B_SPLINE_SURFACE_WITH_KNOTS ( 'NONE', 3, 1, ( 
 ( #21512, #14350 ),
 ( #9830, #23862 ),
 ( #14188, #12172 ),
 ( #23693, #23544 ),
 ( #2505, #12021 ),
 ( #16534, #28706 ),
 ( #21368, #21670 ),
 ( #7344, #306 ),
 ( #7, #19343 ),
 ( #28865, #7498 ),
 ( #16995, #24325 ) ),
 .UNSPECIFIED., .F., .F., .F.,
 ( 4, 1, 1, 1, 1, 1, 1, 1, 4 ),
 ( 2, 2 ),
 ( 0.000000000000000000, 0.3926990816987241395, 0.7853981633974482790, 1.178097245096172418, 1.570796326794896558, 1.963495408493620697, 2.356194490192344837, 2.748893571891068976, 3.141592653589793116 ),
 ( 0.000000000000000000, 1.000000000000000000 ),
 .UNSPECIFIED. ) ;
#10644=CARTESIAN_POINT ( 'NONE',  ( -24.03057240117690441, -26.57182937991348481, 24.50000000000000000 ) ) ;
#10652=CARTESIAN_POINT ( 'NONE',  ( 3.395021109945021376, 30.50000000000000000, 1.500000000000000000 ) ) ;
#10735=ADVANCED_FACE ( 'NONE', ( #19056 ), #5020, .F. ) ;
#10741=CARTESIAN_POINT ( 'NONE',  ( 3.581105043790427711, 42.33170517314361092, 19.86130596537937976 ) ) ;
#10814=CARTESIAN_POINT ( 'NONE',  ( -36.99049879904470117, 13.48014611408327923, 9.989536694329901323 ) ) ;
#10833=ORIENTED_EDGE ( 'NONE', *, *, #617, .T. ) ;
#10924=ORIENTED_EDGE ( 'NONE', *, *, #12401, .T. ) ;
#10929=CARTESIAN_POINT ( 'NONE',  ( -27.75715622479468081, 2.303929616531696922E-16, 1.500000000000000000 ) ) ;
#10948=ORIENTED_EDGE ( 'NONE', *, *, #14165, .F. ) ;
#10969=ORIENTED_EDGE ( 'NONE', *, *, #18537, .F. ) ;
#11022=ORIENTED_EDGE ( 'NONE', *, *, #22530, .T. ) ;
#11114=CARTESIAN_POINT ( 'NONE',  ( 48.64405085385531180, 18.29172496293574213, 24.50000000000000355 ) ) ;
#11142=ORIENTED_EDGE ( 'NONE', *, *, #2132, .F. ) ;
#11186=CARTESIAN_POINT ( 'NONE',  ( -24.03057240117691862, 26.57182937991348481, 24.50000000000000000 ) ) ;
#11208=ORIENTED_EDGE ( 'NONE', *, *, #12202, .F. ) ;
#11229=EDGE_LOOP ( 'NONE', ( #10178, #14081, #10156, #25304, #67, #2123 ) ) ;
#11230=CIRCLE ( 'NONE', #28671, 1.447898107987198646 ) ;
#11275=CARTESIAN_POINT ( 'NONE',  ( -3.469446951953614189E-15, -30.50000000000000711, 24.50000000000000000 ) ) ;
#11390=AXIS2_PLACEMENT_3D ( 'NONE', #8330, #7864, #5983 ) ;
#11400=ORIENTED_EDGE ( 'NONE', *, *, #25059, .F. ) ;
#11407=CARTESIAN_POINT ( 'NONE',  ( 32.87304123117094434, -22.86929295230439152, 18.00000000000000355 ) ) ;
#11420=VECTOR ( 'NONE', #27874, 1000.000000000000000 ) ;
#11431=CARTESIAN_POINT ( 'NONE',  ( 77.99999999999998579, 42.50000000000000711, 1.500000000000001110 ) ) ;
#11432=CARTESIAN_POINT ( 'NONE',  ( -3.576392677004104570, -42.36439329621270389, 19.83430273327883953 ) ) ;
#11440=CARTESIAN_POINT ( 'NONE',  ( 22.58267429318971864, 26.57182937991349903, 1.500000000000001332 ) ) ;
#11442=ORIENTED_EDGE ( 'NONE', *, *, #8452, .T. ) ;
#11489=LINE ( 'NONE', #16315, #11420 ) ;
#11509=( BOUNDED_CURVE ( )  B_SPLINE_CURVE ( 3, ( #24586, #3228, #12751, #4150 ),
 .UNSPECIFIED., .F., .T. ) 
 B_SPLINE_CURVE_WITH_KNOTS ( ( 4, 4 ),
 ( 0.5278016404580625487, 2.613791013131731233 ),
 .UNSPECIFIED. ) 
 CURVE ( )  GEOMETRIC_REPRESENTATION_ITEM ( )  RATIONAL_B_SPLINE_CURVE ( ( 1.000000000000000000, 0.6690902406732673890, 0.6690902406732673890, 1.000000000000000000 ) ) 
 REPRESENTATION_ITEM ( '' )  );
#11510=CARTESIAN_POINT ( 'NONE',  ( 0.000000000000000000, 42.50000000000000000, 1.500000000000000000 ) ) ;
#11517=DIRECTION ( 'NONE',  ( -0.000000000000000000, 1.000000000000000000, -0.000000000000000000 ) ) ;
#11556=FACE_BOUND ( 'NONE', #23613, .T. ) ;
#11610=LINE ( 'NONE', #28313, #29735 ) ;
#11623=CARTESIAN_POINT ( 'NONE',  ( 18.25545825136821421, 37.59715331615011991, 23.77245749941748798 ) ) ;
#11708=EDGE_CURVE ( 'NONE', #26722, #23884, #26573, .T. ) ;
#11766=ORIENTED_EDGE ( 'NONE', *, *, #25026, .T. ) ;
#11781=DIRECTION ( 'NONE',  ( -1.000000000000000000, 0.000000000000000000, 0.000000000000000000 ) ) ;
#11859=CARTESIAN_POINT ( 'NONE',  ( -4.776122516674677878E-15, -42.50000000000000000, 24.50000000000000000 ) ) ;
#11869=FACE_OUTER_BOUND ( 'NONE', #16388, .T. ) ;
#11897=CIRCLE ( 'NONE', #17368, 4.999999999999997335 ) ;
#11925=PRODUCT_DEFINITION_SHAPE ( 'NONE', 'NONE',  #6845 ) ;
#11942=AXIS2_PLACEMENT_3D ( 'NONE', #3482, #22487, #1134 ) ;
#12007=EDGE_CURVE ( 'NONE', #8550, #24015, #8458, .T. ) ;
#12011=CIRCLE ( 'NONE', #21459, 1.447898107987198646 ) ;
#12021=CARTESIAN_POINT ( 'NONE',  ( -25.48568755041063838, 12.36160011285429583, 1.500000000000001332 ) ) ;
#12045=CARTESIAN_POINT ( 'NONE',  ( 24.03057240117690441, -26.57182937991349903, 26.54355021145562787 ) ) ;
#12115=CARTESIAN_POINT ( 'NONE',  ( -77.99999999999998579, -42.49999999999998579, 1.500000000000000222 ) ) ;
#12126=CARTESIAN_POINT ( 'NONE',  ( 36.00889349845778042, -16.33510104555887921, 16.99424500426727036 ) ) ;
#12146=VERTEX_POINT ( 'NONE', #19506 ) ;
#12157=DIRECTION ( 'NONE',  ( -0.000000000000000000, -0.000000000000000000, -1.000000000000000000 ) ) ;
#12160=CARTESIAN_POINT ( 'NONE',  ( -28.29426732178171378, 29.25030496633768706, 11.22274459460341234 ) ) ;
#12172=CARTESIAN_POINT ( 'NONE',  ( -10.18506332983503704, 29.04537757311073776, 1.500000000000001332 ) ) ;
#12173=EDGE_LOOP ( 'NONE', ( #21910, #26795 ) ) ;
#12202=EDGE_CURVE ( 'NONE', #19224, #12146, #15433, .T. ) ;
#12227=ADVANCED_FACE ( 'NONE', ( #3912 ), #8407, .T. ) ;
#12252=AXIS2_PLACEMENT_3D ( 'NONE', #15488, #22361, #20331 ) ;
#12276=DIRECTION ( 'NONE',  ( -0.000000000000000000, -0.000000000000000000, -1.000000000000000000 ) ) ;
#12278=CARTESIAN_POINT ( 'NONE',  ( 37.85012425400401526, -10.24638405728790680, 11.80728464478693240 ) ) ;
#12316=CARTESIAN_POINT ( 'NONE',  ( -29.19944802842337950, 28.17413647968741586, 9.732408078920970596 ) ) ;
#12322=SHAPE_REPRESENTATION ( 'Cam Ring Elliptical Outer Ring', ( #7396 ), #1419 ) ;
#12381=ORIENTED_EDGE ( 'NONE', *, *, #7688, .F. ) ;
#12396=FACE_BOUND ( 'NONE', #9665, .T. ) ;
#12401=EDGE_CURVE ( 'NONE', #27073, #24015, #25720, .T. ) ;
#12426=ORIENTED_EDGE ( 'NONE', *, *, #7245, .F. ) ;
#12470=EDGE_LOOP ( 'NONE', ( #6555, #29439, #14514 ) ) ;
#12478=DIRECTION ( 'NONE',  ( 0.000000000000000000, 0.000000000000000000, 1.000000000000000000 ) ) ;
#12482=CARTESIAN_POINT ( 'NONE',  ( -28.22318188663881600, 29.33129562425243009, 14.53116935034356061 ) ) ;
#12520=CARTESIAN_POINT ( 'NONE',  ( 29.41946586498233529, -27.90099047827807510, 9.493481885648451524 ) ) ;
#12549=FACE_OUTER_BOUND ( 'NONE', #4346, .T. ) ;
#12592=CARTESIAN_POINT ( 'NONE',  ( 37.98801336486642555, -9.618861032953940793, 13.08357279190622791 ) ) ;
#12661=ADVANCED_FACE ( 'NONE', ( #6789 ), #13678, .F. ) ;
#12676=CARTESIAN_POINT ( 'NONE',  ( 29.91322502737726552, -27.27054877340401973, 9.054183611633645157 ) ) ;
#12706=DIRECTION ( 'NONE',  ( -0.000000000000000000, 1.000000000000000000, -0.000000000000000000 ) ) ;
#12731=B_SPLINE_CURVE_WITH_KNOTS ( 'NONE', 3,
 ( #8678, #8825, #6633, #15997, #16146, #18346, #25664, #30483, #27860, #1956, #20959 ),
 .UNSPECIFIED., .F., .F.,
 ( 4, 1, 1, 1, 1, 1, 1, 1, 4 ),
 ( 3.141592653589793116, 3.534291735288517255, 3.926990816987241395, 4.319689898685965090, 4.712388980384689674, 5.105088062083414258, 5.497787143782137953, 5.890486225480861648, 6.283185307179586232 ),
 .UNSPECIFIED. ) ;
#12751=CARTESIAN_POINT ( 'NONE',  ( -48.64405085385531891, -18.29172496293576700, 24.50000000000000355 ) ) ;
#12780=CARTESIAN_POINT ( 'NONE',  ( -31.07284318477800866, 25.68762719043657583, 8.372895414906505351 ) ) ;
#12790=VERTEX_POINT ( 'NONE', #4915 ) ;
#12806=CARTESIAN_POINT ( 'NONE',  ( 19.18576292979354747, 22.55620591602726677, 1.500000000000001332 ) ) ;
#12827=CARTESIAN_POINT ( 'NONE',  ( 28.85400505702477858, -28.59354210116202211, 15.81854097348012544 ) ) ;
#12848=AXIS2_PLACEMENT_3D ( 'NONE', #6236, #3438, #15742 ) ;
#12856=CARTESIAN_POINT ( 'NONE',  ( -37.97827203760240877, 9.664683007568301676, 12.65335581815688748 ) ) ;
#12914=ORIENTED_EDGE ( 'NONE', *, *, #3881, .F. ) ;
#12961=CARTESIAN_POINT ( 'NONE',  ( 3.469446951953614189E-15, 30.50000000000000000, 1.500000000000001332 ) ) ;
#12981=CARTESIAN_POINT ( 'NONE',  ( 32.04644741952905918, -24.22584960208014948, 8.083507045776100242 ) ) ;
#13061=ORIENTED_EDGE ( 'NONE', *, *, #16965, .F. ) ;
#13134=CARTESIAN_POINT ( 'NONE',  ( 28.54797212025346909, -28.95590790227160483, 10.69245695584030997 ) ) ;
#13144=ORIENTED_EDGE ( 'NONE', *, *, #17753, .T. ) ;
#13149=EDGE_LOOP ( 'NONE', ( #22107, #8974 ) ) ;
#13156=CARTESIAN_POINT ( 'NONE',  ( -37.17124714164319244, 12.87530473911888151, 15.75708911316455918 ) ) ;
#13160=CARTESIAN_POINT ( 'NONE',  ( -3.395021109945016491, -30.50000000000000355, 24.50000000000000000 ) ) ;
#13239=MANIFOLD_SOLID_BREP ( 'CirPattern4', #22286 ) ;
#13266=CARTESIAN_POINT ( 'NONE',  ( -19.18576292979354392, -22.55620591602727742, 1.500000000000000000 ) ) ;
#13271=CARTESIAN_POINT ( 'NONE',  ( 10.18506332983503349, -29.04537757311073420, 24.50000000000000000 ) ) ;
#13273=ORIENTED_EDGE ( 'NONE', *, *, #20978, .F. ) ;
#13513=DIRECTION ( 'NONE',  ( 1.000000000000000000, 0.000000000000000000, 0.000000000000000000 ) ) ;
#13621=EDGE_CURVE ( 'NONE', #20574, #26441, #6426, .T. ) ;
#13629=CARTESIAN_POINT ( 'NONE',  ( -24.03057240117691862, 26.57182937991348481, 1.500000000000001332 ) ) ;
#13639=ORIENTED_EDGE ( 'NONE', *, *, #20251, .T. ) ;
#13678=CYLINDRICAL_SURFACE ( 'NONE', #502, 4.999999999999997335 ) ;
#13682=ORIENTED_EDGE ( 'NONE', *, *, #20978, .T. ) ;
#13685=CARTESIAN_POINT ( 'NONE',  ( -24.03057240117690441, -26.57182937991348481, 1.500000000000001332 ) ) ;
#13715=ORIENTED_EDGE ( 'NONE', *, *, #13621, .F. ) ;
#13719=CARTESIAN_POINT ( 'NONE',  ( 25.47847050916410439, -26.57182937991349903, 24.50000000000000000 ) ) ;
#13753=DIRECTION ( 'NONE',  ( 1.000000000000000000, 0.000000000000000000, 0.000000000000000000 ) ) ;
#13777=B_SPLINE_CURVE_WITH_KNOTS ( 'NONE', 3,
 ( #5207, #29379, #3324, #20011, #24852, #8019, #3489, #22494, #1140, #10652, #17051 ),
 .UNSPECIFIED., .F., .F.,
 ( 4, 1, 1, 1, 1, 1, 1, 1, 4 ),
 ( 3.141592653589793116, 3.534291735288517255, 3.926990816987241395, 4.319689898685965090, 4.712388980384689674, 5.105088062083414258, 5.497787143782137953, 5.890486225480861648, 6.283185307179586232 ),
 .UNSPECIFIED. ) ;
#13914=CARTESIAN_POINT ( 'NONE',  ( -4.776122516674677878E-15, -42.50000000000000000, 1.500000000000001332 ) ) ;
#13925=DIRECTION ( 'NONE',  ( -0.000000000000000000, -0.000000000000000000, -1.000000000000000000 ) ) ;
#13964=CARTESIAN_POINT ( 'NONE',  ( 4.473510263713153634, 42.23049256842776344, 19.94491637797075612 ) ) ;
#13971=CARTESIAN_POINT ( 'NONE',  ( 32.98805937973593672, -80.00000000000000000, 13.00000000000000178 ) ) ;
#14081=ORIENTED_EDGE ( 'NONE', *, *, #11708, .T. ) ;
#14140=AXIS2_PLACEMENT_3D ( 'NONE', #5720, #22251, #724 ) ;
#14165=EDGE_CURVE ( 'NONE', #26054, #4436, #6364, .T. ) ;
#14183=CARTESIAN_POINT ( 'NONE',  ( -4.776122516674677878E-15, -42.50000000000000000, 19.72227980406325543 ) ) ;
#14188=CARTESIAN_POINT ( 'NONE',  ( -10.18506332983503704, 29.04537757311073776, 24.50000000000000000 ) ) ;
#14193=ORIENTED_EDGE ( 'NONE', *, *, #2846, .T. ) ;
#14274=CARTESIAN_POINT ( 'NONE',  ( -77.99999999999998579, 42.50000000000000000, 1.500000000000000222 ) ) ;
#14343=FACE_OUTER_BOUND ( 'NONE', #29454, .T. ) ;
#14350=CARTESIAN_POINT ( 'NONE',  ( 2.168404344971008868E-16, 30.50000000000000000, 1.500000000000001332 ) ) ;
#14397=( GEOMETRIC_REPRESENTATION_CONTEXT ( 3 ) GLOBAL_UNCERTAINTY_ASSIGNED_CONTEXT ( ( #4848 ) ) GLOBAL_UNIT_ASSIGNED_CONTEXT ( ( #21403, #7212, #23900 ) ) REPRESENTATION_CONTEXT ( 'NONE', 'WORKASPACE' ) );
#14449=CARTESIAN_POINT ( 'NONE',  ( -4.776122516674677878E-15, -42.50000000000000000, 1.500000000000000000 ) ) ;
#14459=CARTESIAN_POINT ( 'NONE',  ( 36.97777267373784582, -13.52151540233721505, 9.972772046649604150 ) ) ;
#14480=ORIENTED_EDGE ( 'NONE', *, *, #29747, .F. ) ;
#14514=ORIENTED_EDGE ( 'NONE', *, *, #15087, .F. ) ;
#14589=CARTESIAN_POINT ( 'NONE',  ( -24.03057240117690441, -26.57182937991348481, 26.54355021145562787 ) ) ;
#14622=CARTESIAN_POINT ( 'NONE',  ( -19.64177907938615064, 36.71644397333972876, 24.50000000000000000 ) ) ;
#14644=DIRECTION ( 'NONE',  ( -1.000000000000000000, 0.000000000000000000, 0.000000000000000000 ) ) ;
#14647=CARTESIAN_POINT ( 'NONE',  ( -32.53212664356424710, 23.45839305882638470, 8.000000000000005329 ) ) ;
#14682=ORIENTED_EDGE ( 'NONE', *, *, #29747, .T. ) ;
#14704=VERTEX_POINT ( 'NONE', #10445 ) ;
#14756=CARTESIAN_POINT ( 'NONE',  ( 37.41913830146530273, -11.98133940937022146, 15.32185239508652863 ) ) ;
#14765=CARTESIAN_POINT ( 'NONE',  ( -8.832778568892177162, 41.43887595177744032, 20.59886053955145613 ) ) ;
#14840=CARTESIAN_POINT ( 'NONE',  ( 31.80202249548025861, -24.60530730987961689, 8.135760915160240359 ) ) ;
#14884=DIRECTION ( 'NONE',  ( 0.000000000000000000, 0.000000000000000000, 1.000000000000000000 ) ) ;
#14920=LINE ( 'NONE', #19293, #6900 ) ;
#14943=CIRCLE ( 'NONE', #20429, 1.447898107987198646 ) ;
#14978=ORIENTED_EDGE ( 'NONE', *, *, #3881, .T. ) ;
#14994=CARTESIAN_POINT ( 'NONE',  ( 28.22630106158077723, -29.32773264757057419, 11.45922263815823960 ) ) ;
#15018=EDGE_LOOP ( 'NONE', ( #13639, #20510 ) ) ;
#15022=FACE_BOUND ( 'NONE', #20293, .T. ) ;
#15042=CARTESIAN_POINT ( 'NONE',  ( 25.47847050916411504, 26.57182937991349903, 24.50000000000000000 ) ) ;
#15057=ADVANCED_FACE ( 'NONE', ( #7926 ), #8076, .F. ) ;
#15062=CARTESIAN_POINT ( 'NONE',  ( 37.49382109471516600, -11.70052473558270556, 15.17456354887356795 ) ) ;
#15087=EDGE_CURVE ( 'NONE', #24759, #9785, #22833, .T. ) ;
#15127=CARTESIAN_POINT ( 'NONE',  ( 27.75715622479469147, -6.315477654728063328E-15, 24.50000000000000000 ) ) ;
#15145=CARTESIAN_POINT ( 'NONE',  ( 32.98805937973595093, -22.67054169308931222, 8.000000000000003553 ) ) ;
#15204=DIRECTION ( 'NONE',  ( 0.000000000000000000, 0.7709617516270895754, -0.6368814469962912339 ) ) ;
#15245=CARTESIAN_POINT ( 'NONE',  ( -28.86331178595770197, 28.58238193408198313, 10.16794702317896615 ) ) ;
#15265=CARTESIAN_POINT ( 'NONE',  ( 2.168404344971008868E-16, 30.50000000000000000, 1.500000000000000000 ) ) ;
#15272=CARTESIAN_POINT ( 'NONE',  ( 19.18576292979354392, -22.55620591602728453, 24.50000000000000000 ) ) ;
#15279=B_SPLINE_CURVE_WITH_KNOTS ( 'NONE', 3,
 ( #3252, #14647, #26660, #9818, #12780, #22280, #26830, #8105, #2798, #923, #17614, #12316, #27130, #15245, #21821, #24776, #12160, #19331, #463, #28854, #28997, #7634, #5290, #24315, #2966, #12482, #5455, #20106, #1690, #20702, #15894, #3889, #18228, #6380, #27281, #15571, #27905, #18400, #20555, #6062, #22589, #20254 ),
 .UNSPECIFIED., .F., .F.,
 ( 4, 2, 2, 2, 2, 2, 2, 2, 2, 2, 2, 2, 2, 2, 2, 2, 2, 2, 2, 2, 4 ),
 ( 0.000000000000000000, 0.002689500986570608678, 0.004034251479855906729, 0.004706626726498557706, 0.005379001973141206948, 0.006723752466426514973, 0.007396127713069166817, 0.008068502959711818662, 0.009413253452997118881, 0.01008562869963976899, 0.01075800394628241910, 0.01143037919292506921, 0.01210275443956771758, 0.01277512968621036943, 0.01344750493285301780, 0.01479225542613831629, 0.01546463067278096813, 0.01613700591942361651, 0.01748175641270892366, 0.01882650690599423082, 0.02151600789256482779 ),
 .UNSPECIFIED. ) ;
#15296=CARTESIAN_POINT ( 'NONE',  ( 28.06623213401399752, -29.50949589058133071, 13.90928673059489284 ) ) ;
#15314=ORIENTED_EDGE ( 'NONE', *, *, #21525, .F. ) ;
#15365=DIRECTION ( 'NONE',  ( -0.000000000000000000, -1.000000000000000000, -0.000000000000000000 ) ) ;
#15401=DIRECTION ( 'NONE',  ( -0.000000000000000000, -0.000000000000000000, -1.000000000000000000 ) ) ;
#15433=LINE ( 'NONE', #1568, #28370 ) ;
#15483=CARTESIAN_POINT ( 'NONE',  ( -37.39679457499870807, 12.06383856310230307, 10.63618240372393942 ) ) ;
#15488=CARTESIAN_POINT ( 'NONE',  ( 32.98805937973593672, 0.000000000000000000, 13.00000000000000178 ) ) ;
#15552=CARTESIAN_POINT ( 'NONE',  ( -25.47847050916411504, 26.57182937991348481, 1.500000000000001332 ) ) ;
#15554=ORIENTED_EDGE ( 'NONE', *, *, #26543, .T. ) ;
#15570=CARTESIAN_POINT ( 'NONE',  ( -8.074094344234884818E-15, 42.50000000000000000, 19.72227980406325543 ) ) ;
#15571=CARTESIAN_POINT ( 'NONE',  ( -30.29234184432961996, 26.77155622317955164, 17.22256730531661262 ) ) ;
#15675=B_SPLINE_CURVE_WITH_KNOTS ( 'NONE', 3,
 ( #15265, #25106, #24636, #27610, #16167, #10929, #20271, #13266, #1413, #22298, #10608 ),
 .UNSPECIFIED., .F., .F.,
 ( 4, 1, 1, 1, 1, 1, 1, 1, 4 ),
 ( 0.000000000000000000, 0.3926990816987241395, 0.7853981633974482790, 1.178097245096172418, 1.570796326794896558, 1.963495408493620475, 2.356194490192344837, 2.748893571891068976, 3.141592653589793116 ),
 .UNSPECIFIED. ) ;
#15712=LINE ( 'NONE', #909, #29666 ) ;
#15742=DIRECTION ( 'NONE',  ( 1.000000000000000000, 0.000000000000000000, 0.000000000000000000 ) ) ;
#15894=CARTESIAN_POINT ( 'NONE',  ( -29.06468222671494672, 28.34114264639704572, 16.11924918789928185 ) ) ;
#15913=LINE ( 'NONE', #25425, #29271 ) ;
#15947=CARTESIAN_POINT ( 'NONE',  ( -24.03057240117691862, 26.57182937991348481, 1.500000000000001332 ) ) ;
#15970=ORIENTED_EDGE ( 'NONE', *, *, #18756, .F. ) ;
#15990=DIRECTION ( 'NONE',  ( 0.000000000000000000, 0.000000000000000000, 1.000000000000000000 ) ) ;
#15991=CARTESIAN_POINT ( 'NONE',  ( -32.98805937973593672, 0.000000000000000000, 13.00000000000000178 ) ) ;
#15997=CARTESIAN_POINT ( 'NONE',  ( 19.18576292979354392, -22.55620591602728453, 24.50000000000000000 ) ) ;
#16059=EDGE_CURVE ( 'NONE', #16132, #12146, #23137, .T. ) ;
#16082=CARTESIAN_POINT ( 'NONE',  ( 13.73901823217154750, -39.81659909301839662, 21.93900229243933353 ) ) ;
#16112=CYLINDRICAL_SURFACE ( 'NONE', #17277, 1.447898107987198646 ) ;
#16132=VERTEX_POINT ( 'NONE', #5235 ) ;
#16146=CARTESIAN_POINT ( 'NONE',  ( 25.48568755041062062, -12.36160011285429583, 24.50000000000000000 ) ) ;
#16161=ORIENTED_EDGE ( 'NONE', *, *, #22128, .F. ) ;
#16167=CARTESIAN_POINT ( 'NONE',  ( -25.48568755041063838, 12.36160011285429583, 1.500000000000000000 ) ) ;
#16169=CARTESIAN_POINT ( 'NONE',  ( -24.03057240117691862, 26.57182937991348481, 26.54355021145562787 ) ) ;
#16170=VERTEX_POINT ( 'NONE', #15042 ) ;
#16176=VECTOR ( 'NONE', #2854, 1000.000000000000000 ) ;
#16181=DIRECTION ( 'NONE',  ( 0.000000000000000000, 1.000000000000000000, 0.000000000000000000 ) ) ;
#16208=ADVANCED_BREP_SHAPE_REPRESENTATION ( '', ( #13239, #7396 ), #1419 ) ;
#16245=CARTESIAN_POINT ( 'NONE',  ( 77.99999999999998579, -42.50000000000002132, 1.500000000000001110 ) ) ;
#16282=AXIS2_PLACEMENT_3D ( 'NONE', #30583, #23550, #13753 ) ;
#16313=DIRECTION ( 'NONE',  ( 0.000000000000000000, 0.000000000000000000, 1.000000000000000000 ) ) ;
#16315=CARTESIAN_POINT ( 'NONE',  ( 0.000000000000000000, 42.50000000000000000, 24.50000000000000000 ) ) ;
#16343=LINE ( 'NONE', #18994, #26461 ) ;
#16380=CARTESIAN_POINT ( 'NONE',  ( -77.99999999999998579, 42.50000000000000711, 1.500000000000001110 ) ) ;
#16388=EDGE_LOOP ( 'NONE', ( #19392, #27950, #13061, #5278 ) ) ;
#16401=CARTESIAN_POINT ( 'NONE',  ( 0.000000000000000000, 42.50000000000000000, 1.500000000000001332 ) ) ;
#16405=LINE ( 'NONE', #25920, #25293 ) ;
#16446=VERTEX_POINT ( 'NONE', #813 ) ;
#16447=EDGE_CURVE ( 'NONE', #16170, #26054, #21877, .T. ) ;
#16469=ORIENTED_EDGE ( 'NONE', *, *, #16645, .F. ) ;
#16502=SHAPE_REPRESENTATION_RELATIONSHIP ( 'NONE' , 'NONE' ,  #12322, #16208 ) ;
#16504=( BOUNDED_CURVE ( )  B_SPLINE_CURVE ( 3, ( #19818, #26535, #5316, #26686 ),
 .UNSPECIFIED., .F., .T. ) 
 B_SPLINE_CURVE_WITH_KNOTS ( ( 4, 4 ),
 ( 3.141592653589793116, 6.283185307179586232 ),
 .UNSPECIFIED. ) 
 CURVE ( )  GEOMETRIC_REPRESENTATION_ITEM ( )  RATIONAL_B_SPLINE_CURVE ( ( 1.000000000000000000, 0.3333333333333333703, 0.3333333333333333703, 1.000000000000000000 ) ) 
 REPRESENTATION_ITEM ( '' )  );
#16513=EDGE_LOOP ( 'NONE', ( #28986, #21677, #30584, #4913 ) ) ;
#16534=CARTESIAN_POINT ( 'NONE',  ( -27.75715622479468081, 2.303929616531696922E-16, 24.50000000000000000 ) ) ;
#16555=ORIENTED_EDGE ( 'NONE', *, *, #20251, .F. ) ;
#16589=CARTESIAN_POINT ( 'NONE',  ( -33.62559477039935985, 21.53957619641537491, 17.96845262558712975 ) ) ;
#16600=DIRECTION ( 'NONE',  ( 0.000000000000000000, 0.000000000000000000, 1.000000000000000000 ) ) ;
#16633=ORIENTED_EDGE ( 'NONE', *, *, #12007, .T. ) ;
#16645=EDGE_CURVE ( 'NONE', #19224, #17270, #4238, .T. ) ;
#16648=CARTESIAN_POINT ( 'NONE',  ( 32.98805937973592961, -22.67054169308934064, 18.00000000000000000 ) ) ;
#16661=FACE_BOUND ( 'NONE', #3016, .T. ) ;
#16680=VERTEX_POINT ( 'NONE', #30580 ) ;
#16719=ORIENTED_EDGE ( 'NONE', *, *, #24819, .T. ) ;
#16782=EDGE_CURVE ( 'NONE', #29877, #14704, #11230, .T. ) ;
#16793=CIRCLE ( 'NONE', #12848, 1.447898107987198646 ) ;
#16867=EDGE_LOOP ( 'NONE', ( #24005, #9008, #13273, #18808 ) ) ;
#16881=ORIENTED_EDGE ( 'NONE', *, *, #26402, .T. ) ;
#16930=SHAPE_DEFINITION_REPRESENTATION ( #11925, #12322 ) ;
#16951=CARTESIAN_POINT ( 'NONE',  ( 33.63479021130299174, -21.55299138689128213, 8.000000000000007105 ) ) ;
#16963=DIRECTION ( 'NONE',  ( 1.000000000000000000, 0.000000000000000000, -0.000000000000000000 ) ) ;
#16965=EDGE_CURVE ( 'NONE', #23272, #10393, #15675, .T. ) ;
#16973=EDGE_LOOP ( 'NONE', ( #11142, #11022, #664, #28312 ) ) ;
#16995=CARTESIAN_POINT ( 'NONE',  ( 8.539720164285627899E-15, -30.50000000000000711, 24.50000000000000000 ) ) ;
#17026=EDGE_LOOP ( 'NONE', ( #15314, #10969 ) ) ;
#17051=CARTESIAN_POINT ( 'NONE',  ( 2.168404344971008868E-16, 30.50000000000000000, 1.500000000000000000 ) ) ;
#17180=CARTESIAN_POINT ( 'NONE',  ( 29.18339868661345804, -28.19386397657844867, 9.751140820222291339 ) ) ;
#17270=VERTEX_POINT ( 'NONE', #4871 ) ;
#17277=AXIS2_PLACEMENT_3D ( 'NONE', #18467, #13925, #23271 ) ;
#17354=AXIS2_PLACEMENT_3D ( 'NONE', #10039, #10499, #3173 ) ;
#17357=APPLICATION_CONTEXT ( 'automotive_design' ) ;
#17368=AXIS2_PLACEMENT_3D ( 'NONE', #2415, #21734, #16600 ) ;
#17369=CARTESIAN_POINT ( 'NONE',  ( -37.94861706654396727, 9.802039414123830952, 12.35559950699420639 ) ) ;
#17424=DIRECTION ( 'NONE',  ( -0.000000000000000000, -1.000000000000000000, -0.000000000000000000 ) ) ;
#17482=CARTESIAN_POINT ( 'NONE',  ( 3.395021109945009385, -30.50000000000000711, 1.500000000000001332 ) ) ;
#17501=CARTESIAN_POINT ( 'NONE',  ( 32.76094438725117186, -23.06299619967057168, 8.000000000000007105 ) ) ;
#17522=CARTESIAN_POINT ( 'NONE',  ( -34.49515668447323691, 19.83906540583472022, 8.223984938597787675 ) ) ;
#17570=CARTESIAN_POINT ( 'NONE',  ( 36.43862201448670390, -15.16126941994617283, 16.62946957978847351 ) ) ;
#17587=VERTEX_POINT ( 'NONE', #4520 ) ;
#17614=CARTESIAN_POINT ( 'NONE',  ( -29.55668231273981661, 27.73034433992416936, 9.346428711510588627 ) ) ;
#17654=CARTESIAN_POINT ( 'NONE',  ( 31.80160417541173956, -24.60589111005866059, 17.86404149739671965 ) ) ;
#17753=EDGE_CURVE ( 'NONE', #26694, #8742, #15279, .T. ) ;
#17761=CARTESIAN_POINT ( 'NONE',  ( 11.29413195299407491, 40.68967926612123875, 21.21776214944138772 ) ) ;
#17791=CARTESIAN_POINT ( 'NONE',  ( 19.18576292979354747, 22.55620591602726677, 24.50000000000000000 ) ) ;
#17816=CARTESIAN_POINT ( 'NONE',  ( 29.07478158690974013, -28.32671550006340055, 16.11782540859593382 ) ) ;
#17836=CARTESIAN_POINT ( 'NONE',  ( 2.168404344971008868E-16, 30.50000000000000000, 24.50000000000000000 ) ) ;
#17922=AXIS2_PLACEMENT_3D ( 'NONE', #28519, #23822, #16963 ) ;
#17925=CARTESIAN_POINT ( 'NONE',  ( 25.47847050916410439, -26.57182937991349903, 1.500000000000001332 ) ) ;
#17991=UNCERTAINTY_MEASURE_WITH_UNIT (LENGTH_MEASURE( 1.000000000000000082E-05 ), #21477, 'distance_accuracy_value', 'NONE');
#17997=CARTESIAN_POINT ( 'NONE',  ( -18.23283297759883581, -37.58012701748170059, 23.78652270266532653 ) ) ;
#18052=EDGE_LOOP ( 'NONE', ( #21171, #30710, #2939 ) ) ;
#18072=LINE ( 'NONE', #3883, #28480 ) ;
#18128=CIRCLE ( 'NONE', #25537, 4.999999999999997335 ) ;
#18173=ORIENTED_EDGE ( 'NONE', *, *, #16447, .T. ) ;
#18210=FACE_OUTER_BOUND ( 'NONE', #21486, .T. ) ;
#18228=CARTESIAN_POINT ( 'NONE',  ( -29.54217267045739348, 27.74668781839406506, 16.62675390102625528 ) ) ;
#18272=CARTESIAN_POINT ( 'NONE',  ( 19.64177907938615064, -36.71644397333972876, 24.50000000000000000 ) ) ;
#18285=CARTESIAN_POINT ( 'NONE',  ( 22.58267429318970443, -26.57182937991349903, 1.500000000000001332 ) ) ;
#18297=AXIS2_PLACEMENT_3D ( 'NONE', #782, #24811, #29499 ) ;
#18306=FACE_OUTER_BOUND ( 'NONE', #26621, .T. ) ;
#18310=CIRCLE ( 'NONE', #7837, 1.447898107987198646 ) ;
#18346=CARTESIAN_POINT ( 'NONE',  ( 27.75715622479469147, -6.315477654728063328E-15, 24.50000000000000000 ) ) ;
#18351=ADVANCED_FACE ( 'NONE', ( #18907, #28261 ), #3759, .F. ) ;
#18368=DIRECTION ( 'NONE',  ( 0.000000000000000000, 0.000000000000000000, 1.000000000000000000 ) ) ;
#18400=CARTESIAN_POINT ( 'NONE',  ( -31.05590141235049018, 25.71202138535109327, 17.62027412222990819 ) ) ;
#18455=LINE ( 'NONE', #17836, #25967 ) ;
#18464=CARTESIAN_POINT ( 'NONE',  ( -10.18506332983504237, -29.04537757311072710, 24.50000000000000000 ) ) ;
#18467=CARTESIAN_POINT ( 'NONE',  ( -24.03057240117691862, 26.57182937991348481, 26.54355021145562787 ) ) ;
#18502=CARTESIAN_POINT ( 'NONE',  ( 16.80116347819186373, 38.39680910286394777, 23.11187228430608087 ) ) ;
#18537=EDGE_CURVE ( 'NONE', #23884, #28674, #16504, .T. ) ;
#18676=FACE_OUTER_BOUND ( 'NONE', #23818, .T. ) ;
#18705=EDGE_CURVE ( 'NONE', #26694, #26441, #8059, .T. ) ;
#18726=DIRECTION ( 'NONE',  ( -0.000000000000000000, -0.000000000000000000, -1.000000000000000000 ) ) ;
#18756=EDGE_CURVE ( 'NONE', #4436, #26054, #9314, .T. ) ;
#18802=CARTESIAN_POINT ( 'NONE',  ( 19.64177907938615064, 36.71644397333972876, 24.50000000000000000 ) ) ;
#18808=ORIENTED_EDGE ( 'NONE', *, *, #12401, .F. ) ;
#18883=DIRECTION ( 'NONE',  ( -0.000000000000000000, -0.000000000000000000, -1.000000000000000000 ) ) ;
#18907=FACE_BOUND ( 'NONE', #83, .T. ) ;
#18949=CARTESIAN_POINT ( 'NONE',  ( -33.31178504393444229, 22.11114403104716430, 17.99999999999999645 ) ) ;
#18976=EDGE_CURVE ( 'NONE', #4502, #8522, #11610, .T. ) ;
#18994=CARTESIAN_POINT ( 'NONE',  ( 32.98805937973593672, -80.00000000000000000, 8.000000000000003553 ) ) ;
#19000=ORIENTED_EDGE ( 'NONE', *, *, #16965, .T. ) ;
#19005=PLANE ( 'NONE',  #17922 ) ;
#19032=AXIS2_PLACEMENT_3D ( 'NONE', #2217, #23726, #23425 ) ;
#19055=ORIENTED_EDGE ( 'NONE', *, *, #16782, .F. ) ;
#19056=FACE_OUTER_BOUND ( 'NONE', #23057, .T. ) ;
#19073=DIRECTION ( 'NONE',  ( 1.000000000000000000, 0.000000000000000000, 0.000000000000000000 ) ) ;
#19088=CARTESIAN_POINT ( 'NONE',  ( -34.22142550507209080, 20.39476870213973214, 17.85497485759970004 ) ) ;
#19142=ORIENTED_EDGE ( 'NONE', *, *, #10165, .F. ) ;
#19224=VERTEX_POINT ( 'NONE', #1534 ) ;
#19233=CARTESIAN_POINT ( 'NONE',  ( -32.98805937973593672, 22.67054169308932643, 18.00000000000000000 ) ) ;
#19237=DIRECTION ( 'NONE',  ( -1.000000000000000000, 0.000000000000000000, 0.000000000000000000 ) ) ;
#19292=CARTESIAN_POINT ( 'NONE',  ( 37.45985526150776934, -11.82899854519495797, 10.75678081308941003 ) ) ;
#19293=CARTESIAN_POINT ( 'NONE',  ( -32.98805937973593672, 80.00000000000000000, 18.00000000000000000 ) ) ;
#19302=CARTESIAN_POINT ( 'NONE',  ( -13.76736161019652371, 39.80458471794007380, 21.94892721098231902 ) ) ;
#19331=CARTESIAN_POINT ( 'NONE',  ( -28.11661694678904766, 29.45258986749694330, 11.85255554064003647 ) ) ;
#19343=CARTESIAN_POINT ( 'NONE',  ( -10.18506332983503881, -29.04537757311073065, 1.500000000000001332 ) ) ;
#19364=PLANE ( 'NONE',  #4854 ) ;
#19392=ORIENTED_EDGE ( 'NONE', *, *, #799, .T. ) ;
#19393=CARTESIAN_POINT ( 'NONE',  ( -4.776122516674677878E-15, -42.50000000000000000, 24.50000000000000000 ) ) ;
#19446=CARTESIAN_POINT ( 'NONE',  ( 37.95968219450539749, -9.750946698478889729, 13.55336906631367810 ) ) ;
#19506=CARTESIAN_POINT ( 'NONE',  ( -25.47847050916410439, -26.57182937991348481, 1.500000000000001332 ) ) ;
#19515=ORIENTED_EDGE ( 'NONE', *, *, #29806, .T. ) ;
#19526=CARTESIAN_POINT ( 'NONE',  ( 28.00352791766682259, -29.58015274189969901, 12.54700467726770441 ) ) ;
#19557=PLANE ( 'NONE',  #21572 ) ;
#19670=CARTESIAN_POINT ( 'NONE',  ( 32.04552055021039791, -24.22732060750177752, 17.91633598528648719 ) ) ;
#19696=CARTESIAN_POINT ( 'NONE',  ( -35.30770907227059752, 18.09651441509958048, 17.46635781055317338 ) ) ;
#19721=EDGE_LOOP ( 'NONE', ( #19985, #6498, #27719, #8344, #8479, #24623 ) ) ;
#19745=CARTESIAN_POINT ( 'NONE',  ( 37.18355798296265391, -12.83305167619315412, 15.73854473963378098 ) ) ;
#19818=CARTESIAN_POINT ( 'NONE',  ( -4.776122516674677878E-15, -42.50000000000000000, 1.500000000000000000 ) ) ;
#19821=DIRECTION ( 'NONE',  ( 0.000000000000000000, 0.000000000000000000, 1.000000000000000000 ) ) ;
#19834=CARTESIAN_POINT ( 'NONE',  ( 28.84973994773175576, -28.59864475962095653, 10.18777785223225507 ) ) ;
#19862=CARTESIAN_POINT ( 'NONE',  ( -37.16166377660026399, 12.90791798474662500, 10.22883689759567538 ) ) ;
#19881=STYLED_ITEM('',(#30900),#13239);
#19914=EDGE_CURVE ( 'NONE', #8742, #26694, #3970, .T. ) ;
#19918=CARTESIAN_POINT ( 'NONE',  ( 37.94189864131114120, -9.832916137336869866, 12.30666522825201170 ) ) ;
#19973=CARTESIAN_POINT ( 'NONE',  ( 3.395021109945021376, 30.50000000000000000, 24.50000000000000000 ) ) ;
#19979=DIRECTION ( 'NONE',  ( 0.000000000000000000, 0.6368814469962913449, -0.7709617516270896864 ) ) ;
#19985=ORIENTED_EDGE ( 'NONE', *, *, #11708, .F. ) ;
#19991=CARTESIAN_POINT ( 'NONE',  ( 31.30722686493686524, -25.34759660530392367, 17.71607651522528570 ) ) ;
#20011=CARTESIAN_POINT ( 'NONE',  ( 19.18576292979354392, -22.55620591602728453, 1.500000000000000000 ) ) ;
#20106=CARTESIAN_POINT ( 'NONE',  ( -28.45592497607851712, 29.06316056193650965, 15.12214346831152767 ) ) ;
#20125=CARTESIAN_POINT ( 'NONE',  ( -3.469446951953614189E-15, -30.50000000000000711, 24.50000000000000000 ) ) ;
#20144=CARTESIAN_POINT ( 'NONE',  ( 27.98775450039519086, -29.59783709014061515, 12.77861256115351196 ) ) ;
#20163=CARTESIAN_POINT ( 'NONE',  ( -36.61964531808753520, 14.63326766589592154, 9.551232946053056949 ) ) ;
#20251=EDGE_CURVE ( 'NONE', #12146, #16132, #28732, .T. ) ;
#20254=CARTESIAN_POINT ( 'NONE',  ( -32.98805937973593672, 22.67054169308932643, 18.00000000000000000 ) ) ;
#20271=CARTESIAN_POINT ( 'NONE',  ( -25.48568755041063838, -12.36160011285428517, 1.500000000000000000 ) ) ;
#20293=EDGE_LOOP ( 'NONE', ( #5762, #16161 ) ) ;
#20327=CARTESIAN_POINT ( 'NONE',  ( -32.98805937973593672, 0.000000000000000000, 8.000000000000003553 ) ) ;
#20328=CARTESIAN_POINT ( 'NONE',  ( -37.93416654086659889, 9.868537071680707484, 13.74336834489238868 ) ) ;
#20331=DIRECTION ( 'NONE',  ( 0.000000000000000000, 0.000000000000000000, 1.000000000000000000 ) ) ;
#20429=AXIS2_PLACEMENT_3D ( 'NONE', #5150, #7349, #26207 ) ;
#20476=CARTESIAN_POINT ( 'NONE',  ( -8.773161920692750471, -41.42171262360664485, 20.61303894108385037 ) ) ;
#20510=ORIENTED_EDGE ( 'NONE', *, *, #16059, .T. ) ;
#20555=CARTESIAN_POINT ( 'NONE',  ( -31.31139399731532080, 25.34153631408518592, 17.71763994997926162 ) ) ;
#20574=VERTEX_POINT ( 'NONE', #5853 ) ;
#20575=ORIENTED_EDGE ( 'NONE', *, *, #25059, .T. ) ;
#20620=CARTESIAN_POINT ( 'NONE',  ( -1.803040912908196569, -42.50000000000000000, 19.72227980406325898 ) ) ;
#20655=EDGE_CURVE ( 'NONE', #25535, #16170, #25743, .T. ) ;
#20677=CARTESIAN_POINT ( 'NONE',  ( -32.98805937973593672, 0.000000000000000000, 13.00000000000000178 ) ) ;
#20697=PLANE ( 'NONE',  #9772 ) ;
#20702=CARTESIAN_POINT ( 'NONE',  ( -28.84291104180498522, 28.60802559109908216, 15.82428390531839035 ) ) ;
#20811=AXIS2_PLACEMENT_3D ( 'NONE', #21498, #12157, #14644 ) ;
#20813=CARTESIAN_POINT ( 'NONE',  ( 24.03057240117691862, 26.57182937991349903, 1.500000000000001332 ) ) ;
#20823=CARTESIAN_POINT ( 'NONE',  ( 7.103144483462522807, 41.83363135865116789, 20.27275824691663431 ) ) ;
#20959=CARTESIAN_POINT ( 'NONE',  ( 2.168404344971008868E-16, 30.50000000000000000, 24.50000000000000000 ) ) ;
#20978=EDGE_CURVE ( 'NONE', #24015, #8550, #16793, .T. ) ;
#21011=EDGE_CURVE ( 'NONE', #21045, #8550, #15913, .T. ) ;
#21014=DIRECTION ( 'NONE',  ( 1.000000000000000000, 0.000000000000000000, 0.000000000000000000 ) ) ;
#21045=VERTEX_POINT ( 'NONE', #13719 ) ;
#21046=CARTESIAN_POINT ( 'NONE',  ( -77.99999999999998579, 42.50000000000000711, 24.50000000000000000 ) ) ;
#21049=LINE ( 'NONE', #9211, #7660 ) ;
#21054=DIRECTION ( 'NONE',  ( 1.000000000000000000, 0.000000000000000000, 0.000000000000000000 ) ) ;
#21171=ORIENTED_EDGE ( 'NONE', *, *, #18976, .T. ) ;
#21273=CIRCLE ( 'NONE', #24784, 1.447898107987198646 ) ;
#21327=FACE_BOUND ( 'NONE', #15018, .T. ) ;
#21359=CYLINDRICAL_SURFACE ( 'NONE', #1865, 1.447898107987198646 ) ;
#21368=CARTESIAN_POINT ( 'NONE',  ( -25.48568755041063838, -12.36160011285428517, 24.50000000000000000 ) ) ;
#21403=( LENGTH_UNIT ( ) NAMED_UNIT ( * ) SI_UNIT ( .MILLI., .METRE. ) );
#21441=ORIENTED_EDGE ( 'NONE', *, *, #9162, .F. ) ;
#21459=AXIS2_PLACEMENT_3D ( 'NONE', #7782, #12478, #7952 ) ;
#21477=( LENGTH_UNIT ( ) NAMED_UNIT ( * ) SI_UNIT ( .MILLI., .METRE. ) );
#21486=EDGE_LOOP ( 'NONE', ( #12914, #19515, #30026, #9718 ) ) ;
#21490=EDGE_LOOP ( 'NONE', ( #13682, #16633 ) ) ;
#21498=CARTESIAN_POINT ( 'NONE',  ( -24.03057240117690441, -26.57182937991348481, 26.54355021145562787 ) ) ;
#21505=CARTESIAN_POINT ( 'NONE',  ( -77.99999999999998579, -42.49999999999998579, 24.50000000000000000 ) ) ;
#21512=CARTESIAN_POINT ( 'NONE',  ( 2.168404344971008868E-16, 30.50000000000000000, 24.50000000000000000 ) ) ;
#21514=AXIS2_PLACEMENT_3D ( 'NONE', #13629, #22814, #1753 ) ;
#21525=EDGE_CURVE ( 'NONE', #28674, #23884, #25069, .T. ) ;
#21533=CARTESIAN_POINT ( 'NONE',  ( -32.98805937973593672, 22.67054169308932288, 8.000000000000003553 ) ) ;
#21538=DIRECTION ( 'NONE',  ( -0.000000000000000000, -0.000000000000000000, -1.000000000000000000 ) ) ;
#21572=AXIS2_PLACEMENT_3D ( 'NONE', #24387, #3031, #680 ) ;
#21627=CARTESIAN_POINT ( 'NONE',  ( 37.98873790226522118, -9.615455971224255549, 13.00203930632523353 ) ) ;
#21670=CARTESIAN_POINT ( 'NONE',  ( -25.48568755041063838, -12.36160011285428517, 1.500000000000001332 ) ) ;
#21677=ORIENTED_EDGE ( 'NONE', *, *, #2381, .T. ) ;
#21685=CARTESIAN_POINT ( 'NONE',  ( 24.03057240117690441, -26.57182937991349903, 24.50000000000000000 ) ) ;
#21734=DIRECTION ( 'NONE',  ( 0.000000000000000000, 1.000000000000000000, 0.000000000000000000 ) ) ;
#21780=CARTESIAN_POINT ( 'NONE',  ( -39.00000000000000000, 46.58316968839002925, 16.34922658321931976 ) ) ;
#21781=CARTESIAN_POINT ( 'NONE',  ( 37.81968897652127026, -10.37739785557808680, 14.29161961893967181 ) ) ;
#21821=CARTESIAN_POINT ( 'NONE',  ( -28.75875294368007928, 28.70714236740944258, 10.32584181054939165 ) ) ;
#21877=LINE ( 'NONE', #24201, #16176 ) ;
#21896=FACE_OUTER_BOUND ( 'NONE', #16973, .T. ) ;
#21910=ORIENTED_EDGE ( 'NONE', *, *, #18756, .T. ) ;
#21934=CARTESIAN_POINT ( 'NONE',  ( 35.76324912335250161, -16.99827115821247858, 8.803654662221047644 ) ) ;
#22012=CARTESIAN_POINT ( 'NONE',  ( 29.79020748929575291, -27.43254185190355443, 16.85628874541750477 ) ) ;
#22037=CARTESIAN_POINT ( 'NONE',  ( -37.40739136233791129, 12.02481294536538847, 15.34406802053112706 ) ) ;
#22043=FACE_BOUND ( 'NONE', #29484, .T. ) ;
#22082=CARTESIAN_POINT ( 'NONE',  ( 37.63480807633214198, -11.15005181301510362, 14.85427662740586463 ) ) ;
#22107=ORIENTED_EDGE ( 'NONE', *, *, #799, .F. ) ;
#22128=EDGE_CURVE ( 'NONE', #16170, #25535, #22828, .T. ) ;
#22168=CARTESIAN_POINT ( 'NONE',  ( 32.52553806410312376, -23.45536643706434532, 8.015563212847093055 ) ) ;
#22180=CARTESIAN_POINT ( 'NONE',  ( 24.03057240117691862, 26.57182937991349903, 1.500000000000001332 ) ) ;
#22242=CARTESIAN_POINT ( 'NONE',  ( 35.28464582062836996, -18.14901843200646425, 8.522369028210444952 ) ) ;
#22251=DIRECTION ( 'NONE',  ( -0.000000000000000000, -0.000000000000000000, -1.000000000000000000 ) ) ;
#22267=ORIENTED_EDGE ( 'NONE', *, *, #12007, .F. ) ;
#22280=CARTESIAN_POINT ( 'NONE',  ( -30.69494854373527915, 26.21875054186513054, 8.554645101623277625 ) ) ;
#22283=ORIENTED_EDGE ( 'NONE', *, *, #25507, .T. ) ;
#22286=CLOSED_SHELL ( 'NONE', ( #5204, #12661, #15057, #7641, #4429, #9409, #23119, #18351, #787, #23423, #9394, #12227, #6, #5032, #5730, #24703, #1200, #10735, #29375, #3701, #8471, #29010 ) ) ;
#22298=CARTESIAN_POINT ( 'NONE',  ( -3.395021109945016491, -30.50000000000000355, 1.500000000000000000 ) ) ;
#22361=DIRECTION ( 'NONE',  ( 0.000000000000000000, 1.000000000000000000, 0.000000000000000000 ) ) ;
#22432=CARTESIAN_POINT ( 'NONE',  ( 2.168404344971008868E-16, 30.50000000000000000, 24.50000000000000000 ) ) ;
#22487=DIRECTION ( 'NONE',  ( 0.000000000000000000, 0.000000000000000000, 1.000000000000000000 ) ) ;
#22494=CARTESIAN_POINT ( 'NONE',  ( 19.18576292979354747, 22.55620591602726677, 1.500000000000000000 ) ) ;
#22495=CARTESIAN_POINT ( 'NONE',  ( -37.68080749674851404, 10.96349481065684017, 11.26294974525756132 ) ) ;
#22519=ORIENTED_EDGE ( 'NONE', *, *, #4207, .T. ) ;
#22530=EDGE_CURVE ( 'NONE', #24759, #8522, #11509, .T. ) ;
#22578=VECTOR ( 'NONE', #12706, 1000.000000000000000 ) ;
#22585=EDGE_CURVE ( 'NONE', #9785, #28674, #11489, .T. ) ;
#22589=CARTESIAN_POINT ( 'NONE',  ( -32.53389886252318774, 23.45533066602934724, 17.99999999999999645 ) ) ;
#22605=B_SPLINE_CURVE_WITH_KNOTS ( 'NONE', 3,
 ( #15145, #17501, #22168, #12981, #14840, #1278, #8147, #24355, #3151, #12676, #1119, #3002, #12520, #17180, #10318, #19834, #10631, #13134, #24826, #24661, #14994, #29359, #22628, #19526, #20144, #7682, #29191, #15296, #7998, #27171, #5332, #27021, #10478, #29661, #12827, #17816, #29039, #26702, #22012, #969, #27329, #26870, #647, #10162, #19991, #17654, #19670, #7831, #5493, #24506, #11407, #25129 ),
 .UNSPECIFIED., .F., .F.,
 ( 4, 2, 2, 2, 2, 2, 2, 2, 2, 2, 2, 2, 2, 2, 2, 2, 2, 2, 2, 2, 2, 2, 2, 2, 2, 4 ),
 ( 0.03093351381247303605, 0.03229139417284349750, 0.03364927453321395895, 0.03500715489358443427, 0.03636503525395490266, 0.03704397543414014726, 0.03772291561432539186, 0.03840185579451063647, 0.03908079597469588107, 0.03975973615488111873, 0.04043867633506636333, 0.04111761651525160793, 0.04179655669543684560, 0.04247549687562209020, 0.04315443705580733480, 0.04383337723599257940, 0.04451231741617782400, 0.04519125759636306167, 0.04587019777654829933, 0.04722807813691876078, 0.04790701831710400538, 0.04858595849728923610, 0.04994383885765971143, 0.05130171921803017288, 0.05198065939821540360, 0.05265959957840063432 ),
 .UNSPECIFIED. ) ;
#22628=CARTESIAN_POINT ( 'NONE',  ( 28.06446820126206987, -29.51148668445827283, 12.10055096529683638 ) ) ;
#22648=CARTESIAN_POINT ( 'NONE',  ( -37.85956889627766486, 10.20476609408173552, 11.84522522745651862 ) ) ;
#22716=DIRECTION ( 'NONE',  ( 0.000000000000000000, 0.000000000000000000, 1.000000000000000000 ) ) ;
#22733=DIRECTION ( 'NONE',  ( -0.000000000000000000, -1.000000000000000000, -0.000000000000000000 ) ) ;
#22804=ORIENTED_EDGE ( 'NONE', *, *, #1752, .F. ) ;
#22814=DIRECTION ( 'NONE',  ( 0.000000000000000000, 0.000000000000000000, 1.000000000000000000 ) ) ;
#22819=CARTESIAN_POINT ( 'NONE',  ( -19.18576292979354392, -22.55620591602727742, 24.50000000000000000 ) ) ;
#22828=CIRCLE ( 'NONE', #17354, 1.447898107987198646 ) ;
#22833=B_SPLINE_CURVE_WITH_KNOTS ( 'NONE', 3,
 ( #14622, #9787, #29283, #19302, #888, #14765, #3227, #10241, #26797, #24743, #10091, #5574 ),
 .UNSPECIFIED., .F., .F.,
 ( 4, 2, 2, 2, 2, 4 ),
 ( 0.000000000000000000, 0.005323107084052460837, 0.01064621416810492167, 0.01596932125215738338, 0.01863087479418361336, 0.02129242833620984335 ),
 .UNSPECIFIED. ) ;
#22890=CARTESIAN_POINT ( 'NONE',  ( 32.98805937973595093, -22.67054169308931222, 8.000000000000003553 ) ) ;
#22892=CARTESIAN_POINT ( 'NONE',  ( -32.98805937973593672, 80.00000000000000000, 13.00000000000000178 ) ) ;
#22960=CARTESIAN_POINT ( 'NONE',  ( -7.057542262939595190, -41.80922458147114895, 20.29292036719578363 ) ) ;
#22965=CARTESIAN_POINT ( 'NONE',  ( -25.48568755041063838, -12.36160011285428517, 24.50000000000000000 ) ) ;
#23001=CYLINDRICAL_SURFACE ( 'NONE', #23790, 4.999999999999997335 ) ;
#23057=EDGE_LOOP ( 'NONE', ( #7031, #28228, #10924, #22267 ) ) ;
#23119=ADVANCED_FACE ( 'NONE', ( #11869 ), #10633, .T. ) ;
#23137=CIRCLE ( 'NONE', #30138, 1.447898107987198646 ) ;
#23197=( NAMED_UNIT ( * ) PLANE_ANGLE_UNIT ( ) SI_UNIT ( $, .RADIAN. ) );
#23271=DIRECTION ( 'NONE',  ( -1.000000000000000000, 0.000000000000000000, 0.000000000000000000 ) ) ;
#23272=VERTEX_POINT ( 'NONE', #8583 ) ;
#23318=CARTESIAN_POINT ( 'NONE',  ( 13.72236183117461295, 39.79315620192736702, 21.95836815899282612 ) ) ;
#23423=ADVANCED_FACE ( 'NONE', ( #276, #21327, #16661, #2156, #2302, #4961 ), #19005, .F. ) ;
#23425=DIRECTION ( 'NONE',  ( -1.000000000000000000, 0.000000000000000000, 0.000000000000000000 ) ) ;
#23460=CARTESIAN_POINT ( 'NONE',  ( 8.806817561695535090, 41.44469761738502456, 20.59405133752780870 ) ) ;
#23499=EDGE_LOOP ( 'NONE', ( #27599, #11442, #16555, #11208 ) ) ;
#23544=CARTESIAN_POINT ( 'NONE',  ( -19.18576292979354037, 22.55620591602727387, 1.500000000000001332 ) ) ;
#23550=DIRECTION ( 'NONE',  ( 0.000000000000000000, 0.000000000000000000, 1.000000000000000000 ) ) ;
#23613=EDGE_LOOP ( 'NONE', ( #13144, #27156 ) ) ;
#23693=CARTESIAN_POINT ( 'NONE',  ( -19.18576292979354037, 22.55620591602727387, 24.50000000000000000 ) ) ;
#23710=APPLICATION_CONTEXT ( 'automotive_design' ) ;
#23726=DIRECTION ( 'NONE',  ( -0.000000000000000000, -0.000000000000000000, -1.000000000000000000 ) ) ;
#23790=AXIS2_PLACEMENT_3D ( 'NONE', #8826, #1042, #1507 ) ;
#23805=CARTESIAN_POINT ( 'NONE',  ( 35.04158764634705392, -18.66738852729897502, 17.56791008632125184 ) ) ;
#23818=EDGE_LOOP ( 'NONE', ( #14480, #3225 ) ) ;
#23822=DIRECTION ( 'NONE',  ( 0.000000000000000000, 0.000000000000000000, 1.000000000000000000 ) ) ;
#23844=FACE_OUTER_BOUND ( 'NONE', #16513, .T. ) ;
#23862=CARTESIAN_POINT ( 'NONE',  ( -3.395021109945014270, 30.50000000000000355, 1.500000000000001332 ) ) ;
#23884=VERTEX_POINT ( 'NONE', #24842 ) ;
#23900=( NAMED_UNIT ( * ) SI_UNIT ( $, .STERADIAN. ) SOLID_ANGLE_UNIT ( ) );
#23931=DIRECTION ( 'NONE',  ( 1.000000000000000000, 0.000000000000000000, 0.000000000000000000 ) ) ;
#23932=CARTESIAN_POINT ( 'NONE',  ( -24.03057240117690441, -26.57182937991348481, 24.50000000000000000 ) ) ;
#23959=LINE ( 'NONE', #2919, #28203 ) ;
#23960=CARTESIAN_POINT ( 'NONE',  ( -32.98805937973593672, 22.67054169308932643, 18.00000000000000000 ) ) ;
#23961=CARTESIAN_POINT ( 'NONE',  ( 36.40552445234710888, -15.25516137876289591, 9.339579183450858579 ) ) ;
#24005=ORIENTED_EDGE ( 'NONE', *, *, #24082, .T. ) ;
#24015=VERTEX_POINT ( 'NONE', #18285 ) ;
#24038=EDGE_CURVE ( 'NONE', #4502, #6184, #24051, .T. ) ;
#24051=( BOUNDED_CURVE ( )  B_SPLINE_CURVE ( 3, ( #6723, #30284, #11114, #1895 ),
 .UNSPECIFIED., .F., .T. ) 
 B_SPLINE_CURVE_WITH_KNOTS ( ( 4, 4 ),
 ( 3.669394294047855443, 5.755383666721523461 ),
 .UNSPECIFIED. ) 
 CURVE ( )  GEOMETRIC_REPRESENTATION_ITEM ( )  RATIONAL_B_SPLINE_CURVE ( ( 1.000000000000000000, 0.6690902406732677221, 0.6690902406732677221, 1.000000000000000000 ) ) 
 REPRESENTATION_ITEM ( '' )  );
#24082=EDGE_CURVE ( 'NONE', #27073, #21045, #14943, .T. ) ;
#24105=CARTESIAN_POINT ( 'NONE',  ( 0.000000000000000000, 42.50000000000000000, 1.500000000000000000 ) ) ;
#24116=CARTESIAN_POINT ( 'NONE',  ( 37.60209722150239742, -11.28033150005075136, 11.06618368930695340 ) ) ;
#24201=CARTESIAN_POINT ( 'NONE',  ( 25.47847050916411504, 26.57182937991349903, 26.54355021145562787 ) ) ;
#24267=AXIS2_PLACEMENT_3D ( 'NONE', #21780, #417, #15204 ) ;
#24276=CARTESIAN_POINT ( 'NONE',  ( 37.92106016242558297, -9.928229530987605855, 12.17473369872427291 ) ) ;
#24315=CARTESIAN_POINT ( 'NONE',  ( -28.06227104053563082, 29.51396674875200077, 13.88771667678369148 ) ) ;
#24325=CARTESIAN_POINT ( 'NONE',  ( 8.539720164285627899E-15, -30.50000000000000711, 1.500000000000001332 ) ) ;
#24350=VECTOR ( 'NONE', #23931, 1000.000000000000000 ) ;
#24355=CARTESIAN_POINT ( 'NONE',  ( 30.54239299898967630, -26.43236169747734721, 8.629833734104749965 ) ) ;
#24387=CARTESIAN_POINT ( 'NONE',  ( 0.000000000000000000, 0.000000000000000000, 24.50000000000000000 ) ) ;
#24403=PRODUCT_CONTEXT ( 'NONE', #17357, 'mechanical' ) ;
#24428=CARTESIAN_POINT ( 'NONE',  ( 37.98270490079809036, -9.643723784870349647, 13.24503139370895077 ) ) ;
#24506=CARTESIAN_POINT ( 'NONE',  ( 32.75827721992816777, -23.06400683538976892, 17.99609636942189894 ) ) ;
#24516=DIRECTION ( 'NONE',  ( 0.000000000000000000, 0.000000000000000000, 1.000000000000000000 ) ) ;
#24531=CARTESIAN_POINT ( 'NONE',  ( -37.61339438558123049, 11.23552226342446581, 11.09322008216695821 ) ) ;
#24576=CARTESIAN_POINT ( 'NONE',  ( 35.29656769949644257, -18.08766611768221466, 17.44407013695211006 ) ) ;
#24586=CARTESIAN_POINT ( 'NONE',  ( -19.64177907938615064, 36.71644397333972876, 24.50000000000000000 ) ) ;
#24623=ORIENTED_EDGE ( 'NONE', *, *, #21525, .T. ) ;
#24636=CARTESIAN_POINT ( 'NONE',  ( -10.18506332983503704, 29.04537757311073776, 1.500000000000000000 ) ) ;
#24643=CARTESIAN_POINT ( 'NONE',  ( 25.48568755041062417, 12.36160011285428872, 24.50000000000000000 ) ) ;
#24661=CARTESIAN_POINT ( 'NONE',  ( 28.29745255120971947, -29.24632815619922610, 11.25607929549365238 ) ) ;
#24683=CARTESIAN_POINT ( 'NONE',  ( -37.80350513919287891, 10.44985708433032556, 11.63959174695455445 ) ) ;
#24703=ADVANCED_FACE ( 'NONE', ( #18210 ), #28021, .F. ) ;
#24743=CARTESIAN_POINT ( 'NONE',  ( -1.796820731648991254, 42.46605015914154535, 19.75032532477241176 ) ) ;
#24759=VERTEX_POINT ( 'NONE', #8555 ) ;
#24776=CARTESIAN_POINT ( 'NONE',  ( -28.46515462367053928, 29.05384490974418199, 10.83298537692093788 ) ) ;
#24784=AXIS2_PLACEMENT_3D ( 'NONE', #21685, #19821, #29344 ) ;
#24803=CARTESIAN_POINT ( 'NONE',  ( 25.48568755041062062, -12.36160011285429583, 24.50000000000000000 ) ) ;
#24811=DIRECTION ( 'NONE',  ( 0.000000000000000000, 0.000000000000000000, 1.000000000000000000 ) ) ;
#24819=EDGE_CURVE ( 'NONE', #3543, #8417, #12011, .T. ) ;
#24826=CARTESIAN_POINT ( 'NONE',  ( 28.45806911063409927, -29.06066469564322929, 10.87344409778036969 ) ) ;
#24842=CARTESIAN_POINT ( 'NONE',  ( -4.776122516674677878E-15, -42.50000000000000000, 1.500000000000000000 ) ) ;
#24852=CARTESIAN_POINT ( 'NONE',  ( 25.48568755041062062, -12.36160011285429583, 1.500000000000000000 ) ) ;
#24988=VERTEX_POINT ( 'NONE', #22432 ) ;
#25001=CARTESIAN_POINT ( 'NONE',  ( -36.99918769783646155, 13.45200937490941584, 15.99911628778121653 ) ) ;
#25026=EDGE_CURVE ( 'NONE', #3597, #16680, #16343, .T. ) ;
#25059=EDGE_CURVE ( 'NONE', #17587, #3597, #5600, .T. ) ;
#25068=DIRECTION ( 'NONE',  ( -0.000000000000000000, -0.000000000000000000, -1.000000000000000000 ) ) ;
#25069=( BOUNDED_CURVE ( )  B_SPLINE_CURVE ( 3, ( #24105, #14274, #12115, #14449 ),
 .UNSPECIFIED., .F., .T. ) 
 B_SPLINE_CURVE_WITH_KNOTS ( ( 4, 4 ),
 ( 0.000000000000000000, 3.141592653589793116 ),
 .UNSPECIFIED. ) 
 CURVE ( )  GEOMETRIC_REPRESENTATION_ITEM ( )  RATIONAL_B_SPLINE_CURVE ( ( 1.000000000000000000, 0.3333333333333333703, 0.3333333333333333703, 1.000000000000000000 ) ) 
 REPRESENTATION_ITEM ( '' )  );
#25106=CARTESIAN_POINT ( 'NONE',  ( -3.395021109945014270, 30.50000000000000355, 1.500000000000000000 ) ) ;
#25129=CARTESIAN_POINT ( 'NONE',  ( 32.98805937973592961, -22.67054169308934064, 18.00000000000000000 ) ) ;
#25253=( BOUNDED_SURFACE ( )  B_SPLINE_SURFACE ( 3, 1, ( 
 ( #7175, #9513 ),
 ( #21046, #16380 ),
 ( #21505, #25895 ),
 ( #11859, #9207 ) ),
 .UNSPECIFIED., .F., .F., .T. ) 
 B_SPLINE_SURFACE_WITH_KNOTS ( ( 4, 4 ),
 ( 2, 2 ),
 ( 0.000000000000000000, 1.000000000000000000 ),
 ( 0.000000000000000000, 1.000000000000000000 ),
 .UNSPECIFIED. ) 
 GEOMETRIC_REPRESENTATION_ITEM ( )  RATIONAL_B_SPLINE_SURFACE ( (
 ( 1.000000000000000000, 1.000000000000000000),
 ( 0.3333333333333333703, 0.3333333333333333703),
 ( 0.3333333333333333703, 0.3333333333333333703),
 ( 1.000000000000000000, 1.000000000000000000) ) ) 
 REPRESENTATION_ITEM ( '' )  SURFACE ( )  );
#25293=VECTOR ( 'NONE', #9391, 1000.000000000000000 ) ;
#25304=ORIENTED_EDGE ( 'NONE', *, *, #22585, .F. ) ;
#25425=CARTESIAN_POINT ( 'NONE',  ( 25.47847050916410439, -26.57182937991349903, 26.54355021145562787 ) ) ;
#25462=DIRECTION ( 'NONE',  ( 0.000000000000000000, 0.000000000000000000, 1.000000000000000000 ) ) ;
#25475=CARTESIAN_POINT ( 'NONE',  ( -19.64177907938615064, -36.71644397333972876, 24.50000000000000000 ) ) ;
#25507=EDGE_CURVE ( 'NONE', #24988, #23272, #18455, .T. ) ;
#25535=VERTEX_POINT ( 'NONE', #27351 ) ;
#25537=AXIS2_PLACEMENT_3D ( 'NONE', #27211, #27063, #391 ) ;
#25664=CARTESIAN_POINT ( 'NONE',  ( 25.48568755041062417, 12.36160011285428872, 24.50000000000000000 ) ) ;
#25684=DIRECTION ( 'NONE',  ( -1.000000000000000000, 0.000000000000000000, 0.000000000000000000 ) ) ;
#25720=LINE ( 'NONE', #3698, #30857 ) ;
#25743=CIRCLE ( 'NONE', #16282, 1.447898107987198646 ) ;
#25746=AXIS2_PLACEMENT_3D ( 'NONE', #20813, #15990, #13513 ) ;
#25895=CARTESIAN_POINT ( 'NONE',  ( -77.99999999999998579, -42.49999999999998579, 1.500000000000001110 ) ) ;
#25916=CARTESIAN_POINT ( 'NONE',  ( 77.99999999999998579, 42.50000000000000711, 24.50000000000000000 ) ) ;
#25920=CARTESIAN_POINT ( 'NONE',  ( -3.469446951953614189E-15, -30.50000000000000711, 24.50000000000000000 ) ) ;
#25967=VECTOR ( 'NONE', #29677, 1000.000000000000000 ) ;
#26054=VERTEX_POINT ( 'NONE', #9764 ) ;
#26154=CARTESIAN_POINT ( 'NONE',  ( 33.64310889498737822, -21.53861670882606916, 18.00000000000000000 ) ) ;
#26207=DIRECTION ( 'NONE',  ( 1.000000000000000000, 0.000000000000000000, 0.000000000000000000 ) ) ;
#26278=AXIS2_PLACEMENT_3D ( 'NONE', #22180, #24516, #19073 ) ;
#26402=EDGE_CURVE ( 'NONE', #10393, #23272, #13777, .T. ) ;
#26441=VERTEX_POINT ( 'NONE', #20327 ) ;
#26447=FACE_OUTER_BOUND ( 'NONE', #23499, .T. ) ;
#26461=VECTOR ( 'NONE', #11517, 1000.000000000000000 ) ;
#26501=EDGE_CURVE ( 'NONE', #26722, #8522, #8791, .T. ) ;
#26535=CARTESIAN_POINT ( 'NONE',  ( 77.99999999999998579, -42.50000000000001421, 1.500000000000000222 ) ) ;
#26543=EDGE_CURVE ( 'NONE', #14704, #29877, #5038, .T. ) ;
#26573=LINE ( 'NONE', #19393, #6801 ) ;
#26621=EDGE_LOOP ( 'NONE', ( #16719, #14978, #19055, #12426 ) ) ;
#26660=CARTESIAN_POINT ( 'NONE',  ( -32.05716845166662665, 24.22161781167242722, 8.060878346463965727 ) ) ;
#26686=CARTESIAN_POINT ( 'NONE',  ( 0.000000000000000000, 42.50000000000000000, 1.500000000000000000 ) ) ;
#26694=VERTEX_POINT ( 'NONE', #21533 ) ;
#26702=CARTESIAN_POINT ( 'NONE',  ( 29.54401593347832744, -27.74630720509791004, 16.64138351564043461 ) ) ;
#26719=ORIENTED_EDGE ( 'NONE', *, *, #7688, .T. ) ;
#26722=VERTEX_POINT ( 'NONE', #10303 ) ;
#26729=CARTESIAN_POINT ( 'NONE',  ( -32.98805937973593672, 22.67054169308932288, 8.000000000000003553 ) ) ;
#26789=CARTESIAN_POINT ( 'NONE',  ( 37.97387049854970797, -9.685240207147352010, 12.59636151973351659 ) ) ;
#26795=ORIENTED_EDGE ( 'NONE', *, *, #14165, .T. ) ;
#26797=CARTESIAN_POINT ( 'NONE',  ( -3.580889173201297293, 42.33168915099381024, 19.86131920106836546 ) ) ;
#26830=CARTESIAN_POINT ( 'NONE',  ( -30.56823942190705523, 26.39394548910274452, 8.622060075595381790 ) ) ;
#26858=FACE_OUTER_BOUND ( 'NONE', #18052, .T. ) ;
#26870=CARTESIAN_POINT ( 'NONE',  ( 30.55067843133129912, -26.41807869720452473, 17.36820027845536174 ) ) ;
#26943=CARTESIAN_POINT ( 'NONE',  ( 37.97804311825484547, -9.665537939806041479, 13.32538434702631669 ) ) ;
#26992=ORIENTED_EDGE ( 'NONE', *, *, #617, .F. ) ;
#27004=CARTESIAN_POINT ( 'NONE',  ( 10.18506332983503349, -29.04537757311073420, 1.500000000000001332 ) ) ;
#27021=CARTESIAN_POINT ( 'NONE',  ( 28.46402972798047060, -29.05374092982643575, 15.13942714145325041 ) ) ;
#27037=DIRECTION ( 'NONE',  ( -0.000000000000000000, -0.000000000000000000, -1.000000000000000000 ) ) ;
#27043=CARTESIAN_POINT ( 'NONE',  ( -37.47155912781716580, 11.78490175834441267, 10.78014334239690797 ) ) ;
#27063=DIRECTION ( 'NONE',  ( 0.000000000000000000, -1.000000000000000000, 0.000000000000000000 ) ) ;
#27073=VERTEX_POINT ( 'NONE', #4354 ) ;
#27130=CARTESIAN_POINT ( 'NONE',  ( -29.08334023542832369, 28.31627646104946194, 9.871544281921535102 ) ) ;
#27156=ORIENTED_EDGE ( 'NONE', *, *, #19914, .T. ) ;
#27171=CARTESIAN_POINT ( 'NONE',  ( 28.22957482844025989, -29.32399075545982470, 14.55061583020274441 ) ) ;
#27211=CARTESIAN_POINT ( 'NONE',  ( -32.98805937973593672, 0.000000000000000000, 13.00000000000000178 ) ) ;
#27241=CARTESIAN_POINT ( 'NONE',  ( 19.64177907938615064, 36.71644397333972876, 24.50000000000000000 ) ) ;
#27264=ORIENTED_EDGE ( 'NONE', *, *, #20655, .T. ) ;
#27281=CARTESIAN_POINT ( 'NONE',  ( -29.91502160997805149, 27.26821511153454480, 16.94723710781324399 ) ) ;
#27329=CARTESIAN_POINT ( 'NONE',  ( 30.29603128833749537, -26.76406484782719275, 17.21603893666378582 ) ) ;
#27351=CARTESIAN_POINT ( 'NONE',  ( 22.58267429318971864, 26.57182937991349903, 24.50000000000000000 ) ) ;
#27376=EDGE_LOOP ( 'NONE', ( #19142, #22519, #22283, #3358 ) ) ;
#27599=ORIENTED_EDGE ( 'NONE', *, *, #16645, .T. ) ;
#27610=CARTESIAN_POINT ( 'NONE',  ( -19.18576292979354037, 22.55620591602727387, 1.500000000000000000 ) ) ;
#27654=CARTESIAN_POINT ( 'NONE',  ( -16.76805339484686286, -38.38162967533393299, 23.12441181139608659 ) ) ;
#27659=CARTESIAN_POINT ( 'NONE',  ( -10.18506332983503704, 29.04537757311073776, 24.50000000000000000 ) ) ;
#27662=CARTESIAN_POINT ( 'NONE',  ( 19.64177907938615064, -36.71644397333972876, 24.50000000000000000 ) ) ;
#27695=FACE_OUTER_BOUND ( 'NONE', #28229, .T. ) ;
#27719=ORIENTED_EDGE ( 'NONE', *, *, #22530, .F. ) ;
#27762=ORIENTED_EDGE ( 'NONE', *, *, #16447, .F. ) ;
#27795=CARTESIAN_POINT ( 'NONE',  ( 18.25048847709279443, -37.60031054104898374, 23.76984935710975577 ) ) ;
#27828=CYLINDRICAL_SURFACE ( 'NONE', #19032, 1.447898107987198646 ) ;
#27860=CARTESIAN_POINT ( 'NONE',  ( 10.18506332983505303, 29.04537757311072710, 24.50000000000000000 ) ) ;
#27874=DIRECTION ( 'NONE',  ( -0.000000000000000000, -0.000000000000000000, -1.000000000000000000 ) ) ;
#27880=DIRECTION ( 'NONE',  ( 1.000000000000000000, 0.000000000000000000, 0.000000000000000000 ) ) ;
#27884=DIRECTION ( 'NONE',  ( 1.000000000000000000, 0.000000000000000000, 0.000000000000000000 ) ) ;
#27905=CARTESIAN_POINT ( 'NONE',  ( -30.54665521170317888, 26.42654420156934947, 17.37260941130015013 ) ) ;
#27950=ORIENTED_EDGE ( 'NONE', *, *, #10165, .T. ) ;
#27964=CARTESIAN_POINT ( 'NONE',  ( -9.627708240023329367, -41.19544438224844640, 20.79995618394494272 ) ) ;
#28021=CYLINDRICAL_SURFACE ( 'NONE', #5040, 1.447898107987198646 ) ;
#28153=CARTESIAN_POINT ( 'NONE',  ( 0.8981854125223266427, 42.50000000000000711, 19.72227980406324832 ) ) ;
#28203=VECTOR ( 'NONE', #12276, 1000.000000000000000 ) ;
#28228=ORIENTED_EDGE ( 'NONE', *, *, #35, .T. ) ;
#28229=EDGE_LOOP ( 'NONE', ( #12381, #13715 ) ) ;
#28261=FACE_OUTER_BOUND ( 'NONE', #11229, .T. ) ;
#28312=ORIENTED_EDGE ( 'NONE', *, *, #24038, .T. ) ;
#28313=CARTESIAN_POINT ( 'NONE',  ( 0.000000000000000000, -36.71644397333972165, 24.50000000000000000 ) ) ;
#28368=( NAMED_UNIT ( * ) SI_UNIT ( $, .STERADIAN. ) SOLID_ANGLE_UNIT ( ) );
#28370=VECTOR ( 'NONE', #8127, 1000.000000000000000 ) ;
#28424=DIRECTION ( 'NONE',  ( -1.000000000000000000, 0.000000000000000000, 0.000000000000000000 ) ) ;
#28480=VECTOR ( 'NONE', #8568, 1000.000000000000000 ) ;
#28514=DIRECTION ( 'NONE',  ( 0.000000000000000000, 0.000000000000000000, 1.000000000000000000 ) ) ;
#28519=CARTESIAN_POINT ( 'NONE',  ( 0.000000000000000000, 0.000000000000000000, 1.500000000000000000 ) ) ;
#28576=EDGE_CURVE ( 'NONE', #4502, #26722, #1038, .T. ) ;
#28615=B_SPLINE_CURVE_WITH_KNOTS ( 'NONE', 3,
 ( #3646, #8639, #27659, #8948, #1911, #1759, #22965, #22819, #18464, #13160, #11275 ),
 .UNSPECIFIED., .F., .F.,
 ( 4, 1, 1, 1, 1, 1, 1, 1, 4 ),
 ( 0.000000000000000000, 0.3926990816987241395, 0.7853981633974482790, 1.178097245096172418, 1.570796326794896558, 1.963495408493620475, 2.356194490192344837, 2.748893571891068976, 3.141592653589793116 ),
 .UNSPECIFIED. ) ;
#28671=AXIS2_PLACEMENT_3D ( 'NONE', #15947, #25462, #21054 ) ;
#28674=VERTEX_POINT ( 'NONE', #11510 ) ;
#28701=CARTESIAN_POINT ( 'NONE',  ( 3.582389001540554840, -42.36371625716371625, 19.83486202640626672 ) ) ;
#28706=CARTESIAN_POINT ( 'NONE',  ( -27.75715622479468081, 2.303929616531696922E-16, 1.500000000000001332 ) ) ;
#28732=CIRCLE ( 'NONE', #18297, 1.447898107987198646 ) ;
#28811=CARTESIAN_POINT ( 'NONE',  ( 36.60626274880365116, -14.67294879964692278, 9.537266162416086601 ) ) ;
#28854=CARTESIAN_POINT ( 'NONE',  ( -28.00567590795085238, 29.57774132268513512, 12.52310953214416323 ) ) ;
#28865=CARTESIAN_POINT ( 'NONE',  ( -3.395021109945006721, -30.50000000000000711, 24.50000000000000000 ) ) ;
#28962=CARTESIAN_POINT ( 'NONE',  ( 37.98476534559758733, -9.634081485176503534, 12.75486969068182397 ) ) ;
#28986=ORIENTED_EDGE ( 'NONE', *, *, #8452, .F. ) ;
#28997=CARTESIAN_POINT ( 'NONE',  ( -27.98912715346896007, 29.59629564344513142, 12.74957844391862949 ) ) ;
#29010=ADVANCED_FACE ( 'NONE', ( #27695 ), #4135, .F. ) ;
#29039=CARTESIAN_POINT ( 'NONE',  ( 29.19058584261892619, -28.18502476532347600, 16.25721844935590710 ) ) ;
#29179=CARTESIAN_POINT ( 'NONE',  ( -39.00000000000000000, -46.58316968839002925, 16.34922658321931976 ) ) ;
#29191=CARTESIAN_POINT ( 'NONE',  ( 28.00422547688649644, -29.57936985937913477, 13.46106986886504941 ) ) ;
#29221=CARTESIAN_POINT ( 'NONE',  ( -37.81047817032544600, 10.41981227368125218, 14.33565414798128934 ) ) ;
#29271=VECTOR ( 'NONE', #30545, 1000.000000000000000 ) ;
#29283=CARTESIAN_POINT ( 'NONE',  ( -16.80735851984694662, 38.39305298849780002, 23.11497516139116826 ) ) ;
#29336=ORIENTED_EDGE ( 'NONE', *, *, #19914, .F. ) ;
#29344=DIRECTION ( 'NONE',  ( 1.000000000000000000, 0.000000000000000000, 0.000000000000000000 ) ) ;
#29354=CIRCLE ( 'NONE', #9934, 1.447898107987198646 ) ;
#29359=CARTESIAN_POINT ( 'NONE',  ( 28.10944024216546211, -29.46071976086648192, 11.88312378939523306 ) ) ;
#29375=ADVANCED_FACE ( 'NONE', ( #12549 ), #29857, .F. ) ;
#29379=CARTESIAN_POINT ( 'NONE',  ( 3.395021109945009385, -30.50000000000000711, 1.500000000000000222 ) ) ;
#29380=CARTESIAN_POINT ( 'NONE',  ( -36.41962120944751291, 15.21524643282687350, 9.352698495745318752 ) ) ;
#29432=CARTESIAN_POINT ( 'NONE',  ( 37.38490933374808378, -12.10749625520922024, 10.61420996327511723 ) ) ;
#29439=ORIENTED_EDGE ( 'NONE', *, *, #8805, .F. ) ;
#29454=EDGE_LOOP ( 'NONE', ( #27264, #18173, #15970, #1962 ) ) ;
#29484=EDGE_LOOP ( 'NONE', ( #4789, #7368 ) ) ;
#29492=CARTESIAN_POINT ( 'NONE',  ( 3.395021109945021376, 30.50000000000000000, 1.500000000000001332 ) ) ;
#29499=DIRECTION ( 'NONE',  ( 1.000000000000000000, 0.000000000000000000, 0.000000000000000000 ) ) ;
#29532=CARTESIAN_POINT ( 'NONE',  ( -37.86695649773925965, 10.17204804043823962, 14.12367837669096460 ) ) ;
#29588=DIRECTION ( 'NONE',  ( -0.000000000000000000, -0.000000000000000000, -1.000000000000000000 ) ) ;
#29643=CARTESIAN_POINT ( 'NONE',  ( 25.48568755041062062, -12.36160011285429583, 1.500000000000001332 ) ) ;
#29661=CARTESIAN_POINT ( 'NONE',  ( 28.74947044913098892, -28.71817798780287845, 15.65945394955731196 ) ) ;
#29666=VECTOR ( 'NONE', #15401, 1000.000000000000000 ) ;
#29677=DIRECTION ( 'NONE',  ( -0.000000000000000000, -0.000000000000000000, -1.000000000000000000 ) ) ;
#29735=VECTOR ( 'NONE', #19237, 1000.000000000000000 ) ;
#29747=EDGE_CURVE ( 'NONE', #16446, #16680, #11897, .T. ) ;
#29805=CARTESIAN_POINT ( 'NONE',  ( 3.395021109945009385, -30.50000000000000711, 24.50000000000000000 ) ) ;
#29806=EDGE_CURVE ( 'NONE', #8417, #3543, #18310, .T. ) ;
#29853=CARTESIAN_POINT ( 'NONE',  ( -37.92875555959543021, 9.893234292455838741, 12.22166928970610478 ) ) ;
#29857=CYLINDRICAL_SURFACE ( 'NONE', #11390, 4.999999999999997335 ) ;
#29877=VERTEX_POINT ( 'NONE', #15552 ) ;
#29920=ORIENTED_EDGE ( 'NONE', *, *, #16782, .T. ) ;
#29956=CARTESIAN_POINT ( 'NONE',  ( -3.469446951953614189E-15, -30.50000000000000711, 1.500000000000001332 ) ) ;
#30026=ORIENTED_EDGE ( 'NONE', *, *, #7245, .T. ) ;
#30128=DIRECTION ( 'NONE',  ( 0.000000000000000000, 0.000000000000000000, 1.000000000000000000 ) ) ;
#30138=AXIS2_PLACEMENT_3D ( 'NONE', #13685, #18368, #27880 ) ;
#30284=CARTESIAN_POINT ( 'NONE',  ( 48.64405085385529759, -18.29172496293579542, 24.50000000000000355 ) ) ;
#30353=DIRECTION ( 'NONE',  ( -0.000000000000000000, 1.000000000000000000, -0.000000000000000000 ) ) ;
#30357=EDGE_LOOP ( 'NONE', ( #19000, #16881 ) ) ;
#30469=ORIENTED_EDGE ( 'NONE', *, *, #18705, .T. ) ;
#30483=CARTESIAN_POINT ( 'NONE',  ( 19.18576292979354747, 22.55620591602726677, 24.50000000000000000 ) ) ;
#30545=DIRECTION ( 'NONE',  ( -0.000000000000000000, -0.000000000000000000, -1.000000000000000000 ) ) ;
#30580=CARTESIAN_POINT ( 'NONE',  ( 32.98805937973593672, 0.000000000000000000, 8.000000000000003553 ) ) ;
#30583=CARTESIAN_POINT ( 'NONE',  ( 24.03057240117691862, 26.57182937991349903, 24.50000000000000000 ) ) ;
#30584=ORIENTED_EDGE ( 'NONE', *, *, #12202, .T. ) ;
#30600=FACE_OUTER_BOUND ( 'NONE', #9531, .T. ) ;
#30666=DIRECTION ( 'NONE',  ( 0.000000000000000000, -0.000000000000000000, 1.000000000000000000 ) ) ;
#30710=ORIENTED_EDGE ( 'NONE', *, *, #26501, .F. ) ;
#30712=CARTESIAN_POINT ( 'NONE',  ( 24.03057240117691862, 26.57182937991349903, 26.54355021145562787 ) ) ;
#30717=CARTESIAN_POINT ( 'NONE',  ( 1.808288630848430056, -42.50000000000000711, 19.72227980406325898 ) ) ;
#30857=VECTOR ( 'NONE', #29588, 1000.000000000000000 ) ;
#30894=COLOUR_RGB('Grey',0.48,0.52,0.57);
#30895=FILL_AREA_STYLE_COLOUR('',#30894);
#30896=FILL_AREA_STYLE('',(#30895));
#30897=SURFACE_STYLE_FILL_AREA(#30896);
#30898=SURFACE_SIDE_STYLE('',(#30897));
#30899=SURFACE_STYLE_USAGE(.BOTH.,#30898);
#30900=PRESENTATION_STYLE_ASSIGNMENT((#30899));
ENDSEC;
END-ISO-10303-21;
